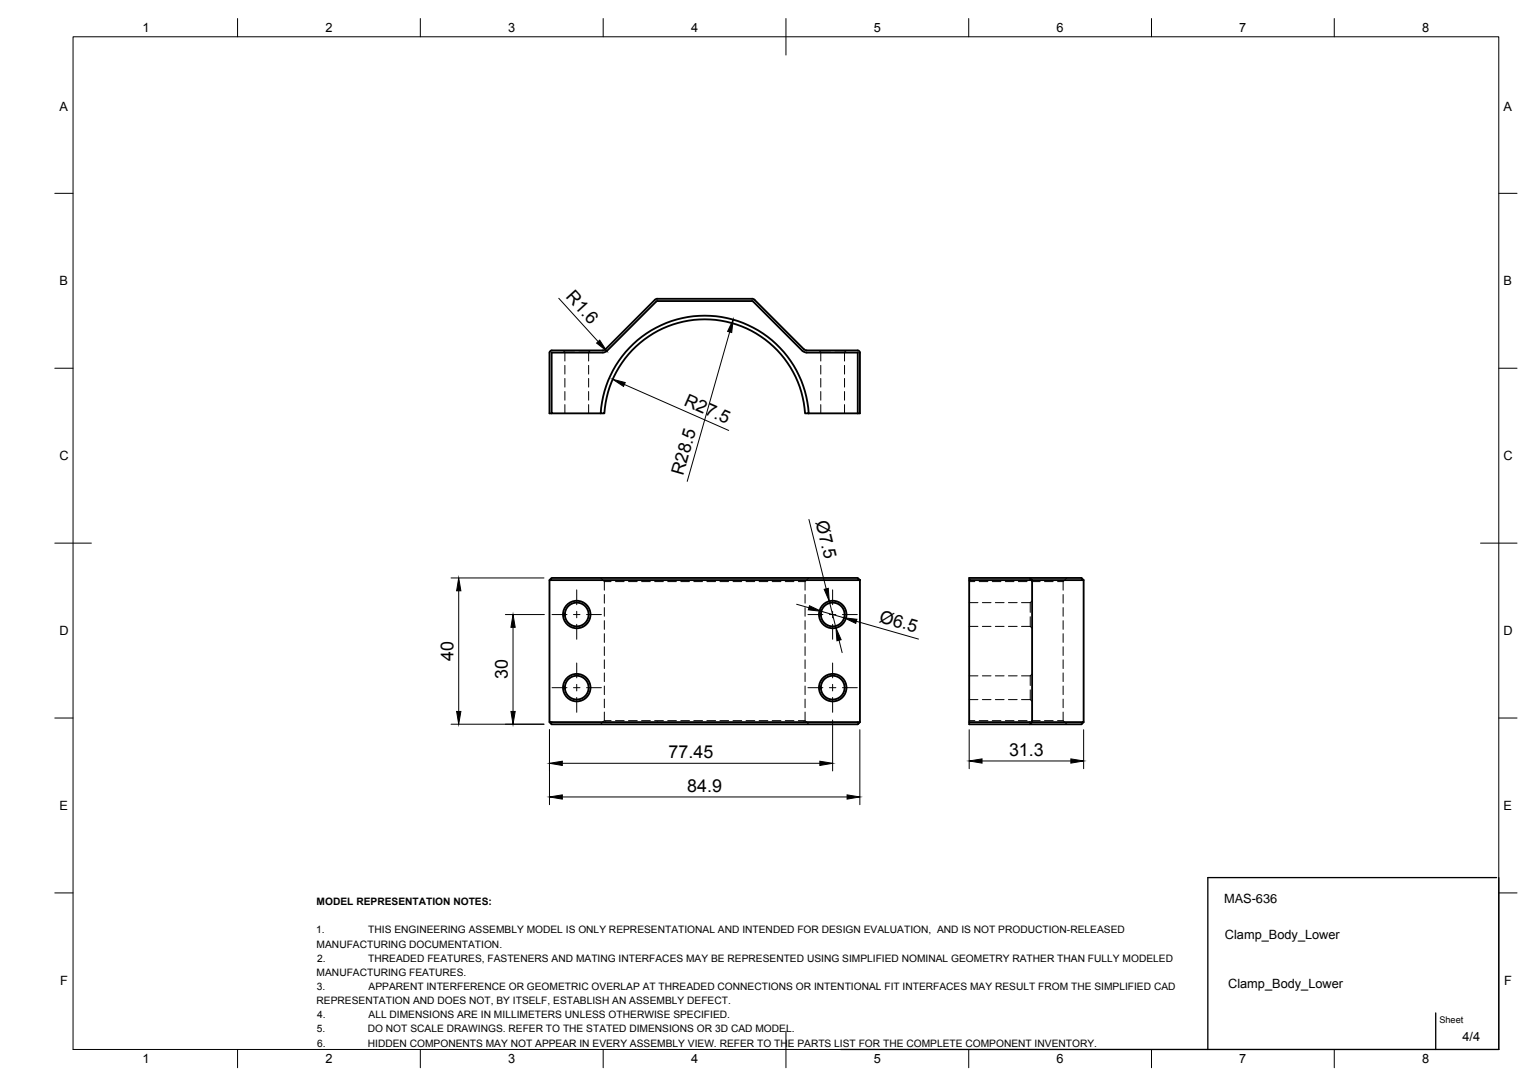
ISO-10303-21;
HEADER;
FILE_DESCRIPTION((''),'2;1');
FILE_NAME('Clamp_Body_Lower.step','2026-10-09T10:15:02-07:00',(''),(''),'','','');
FILE_SCHEMA (('AUTOMOTIVE_DESIGN { 1 0 10303 214 3 1 1 }'));
ENDSEC;
DATA;
#10=MECHANICAL_DESIGN_GEOMETRIC_PRESENTATION_REPRESENTATION('',(#84),#6779);
#59=B_SPLINE_CURVE_WITH_KNOTS('',3,(#6151,#6152,#6153,#6154),
 .UNSPECIFIED.,.F.,.F.,(4,4),(0.,2.0142284459),.UNSPECIFIED.) ;
#60=B_SPLINE_CURVE_WITH_KNOTS('',3,(#6158,#6159,#6160,#6161),
 .UNSPECIFIED.,.F.,.F.,(4,4),(0.,2.0142284459),.UNSPECIFIED.) ;
#61=B_SPLINE_CURVE_WITH_KNOTS('',3,(#6173,#6174,#6175,#6176),
 .UNSPECIFIED.,.F.,.F.,(4,4),(0.,2.0142284459),.UNSPECIFIED.) ;
#62=B_SPLINE_CURVE_WITH_KNOTS('',3,(#6177,#6178,#6179,#6180),
 .UNSPECIFIED.,.F.,.F.,(4,4),(0.,2.0142284459),.UNSPECIFIED.) ;
#64=SHAPE_REPRESENTATION_RELATIONSHIP('SRR','None',#6818,#74) ;
#74=ADVANCED_BREP_SHAPE_REPRESENTATION('',(#94),#6770) ;
#84=STYLED_ITEM('',(#6876),#94) ;
#94=MANIFOLD_SOLID_BREP('Body1',#3896) ;
#111=FACE_BOUND('',#719,.T.) ;
#112=FACE_BOUND('',#720,.T.) ;
#113=FACE_BOUND('',#722,.T.) ;
#114=FACE_BOUND('',#723,.T.) ;
#115=FACE_BOUND('',#745,.T.) ;
#116=FACE_BOUND('',#746,.T.) ;
#117=FACE_BOUND('',#752,.T.) ;
#118=FACE_BOUND('',#753,.T.) ;
#190=PLANE('',#4200) ;
#191=PLANE('',#4209) ;
#192=PLANE('',#4212) ;
#193=PLANE('',#4215) ;
#194=PLANE('',#4218) ;
#195=PLANE('',#4221) ;
#196=PLANE('',#4224) ;
#197=PLANE('',#4225) ;
#198=PLANE('',#4226) ;
#199=PLANE('',#4237) ;
#200=PLANE('',#4238) ;
#201=PLANE('',#4241) ;
#202=PLANE('',#4244) ;
#203=PLANE('',#4247) ;
#204=PLANE('',#4250) ;
#205=PLANE('',#4253) ;
#206=PLANE('',#4257) ;
#207=PLANE('',#4259) ;
#208=PLANE('',#4261) ;
#209=PLANE('',#4263) ;
#210=PLANE('',#4265) ;
#211=PLANE('',#4267) ;
#212=PLANE('',#4268) ;
#213=PLANE('',#4277) ;
#214=PLANE('',#4288) ;
#305=CONICAL_SURFACE('',#4193,1.,0.785398163397) ;
#306=CONICAL_SURFACE('',#4198,1.,0.785398163397) ;
#307=CONICAL_SURFACE('',#4207,1.,0.785398163397) ;
#308=CONICAL_SURFACE('',#4210,1.,0.785398163397) ;
#309=CONICAL_SURFACE('',#4213,1.,0.785398163397) ;
#310=CONICAL_SURFACE('',#4216,1.,0.785398163397) ;
#311=CONICAL_SURFACE('',#4219,1.,0.785398163397) ;
#312=CONICAL_SURFACE('',#4222,1.,0.785398163397) ;
#313=CONICAL_SURFACE('',#4256,1.,0.785398163397) ;
#314=CONICAL_SURFACE('',#4258,1.,0.785398163397) ;
#315=CONICAL_SURFACE('',#4260,1.,0.785398163397) ;
#316=CONICAL_SURFACE('',#4262,1.,0.785398163397) ;
#317=CONICAL_SURFACE('',#4264,1.,0.785398163397) ;
#318=CONICAL_SURFACE('',#4266,1.,0.785398163397) ;
#319=CONICAL_SURFACE('',#4272,1.,0.785398163398) ;
#320=CONICAL_SURFACE('',#4279,1.,0.785398163398) ;
#321=CONICAL_SURFACE('',#4283,1.,0.785398163398) ;
#322=CONICAL_SURFACE('',#4290,1.,0.785398163398) ;
#441=FACE_OUTER_BOUND('',#693,.T.) ;
#442=FACE_OUTER_BOUND('',#694,.T.) ;
#443=FACE_OUTER_BOUND('',#695,.T.) ;
#444=FACE_OUTER_BOUND('',#696,.T.) ;
#445=FACE_OUTER_BOUND('',#697,.T.) ;
#446=FACE_OUTER_BOUND('',#698,.T.) ;
#447=FACE_OUTER_BOUND('',#699,.T.) ;
#448=FACE_OUTER_BOUND('',#700,.T.) ;
#449=FACE_OUTER_BOUND('',#701,.T.) ;
#450=FACE_OUTER_BOUND('',#702,.T.) ;
#451=FACE_OUTER_BOUND('',#703,.T.) ;
#452=FACE_OUTER_BOUND('',#704,.T.) ;
#453=FACE_OUTER_BOUND('',#705,.T.) ;
#454=FACE_OUTER_BOUND('',#706,.T.) ;
#455=FACE_OUTER_BOUND('',#707,.T.) ;
#456=FACE_OUTER_BOUND('',#708,.T.) ;
#457=FACE_OUTER_BOUND('',#709,.T.) ;
#458=FACE_OUTER_BOUND('',#710,.T.) ;
#459=FACE_OUTER_BOUND('',#711,.T.) ;
#460=FACE_OUTER_BOUND('',#712,.T.) ;
#461=FACE_OUTER_BOUND('',#713,.T.) ;
#462=FACE_OUTER_BOUND('',#714,.T.) ;
#463=FACE_OUTER_BOUND('',#715,.T.) ;
#464=FACE_OUTER_BOUND('',#716,.T.) ;
#465=FACE_OUTER_BOUND('',#717,.T.) ;
#466=FACE_OUTER_BOUND('',#718,.T.) ;
#467=FACE_OUTER_BOUND('',#721,.T.) ;
#468=FACE_OUTER_BOUND('',#724,.T.) ;
#469=FACE_OUTER_BOUND('',#725,.T.) ;
#470=FACE_OUTER_BOUND('',#726,.T.) ;
#471=FACE_OUTER_BOUND('',#727,.T.) ;
#472=FACE_OUTER_BOUND('',#728,.T.) ;
#473=FACE_OUTER_BOUND('',#729,.T.) ;
#474=FACE_OUTER_BOUND('',#730,.T.) ;
#475=FACE_OUTER_BOUND('',#731,.T.) ;
#476=FACE_OUTER_BOUND('',#732,.T.) ;
#477=FACE_OUTER_BOUND('',#733,.T.) ;
#478=FACE_OUTER_BOUND('',#734,.T.) ;
#479=FACE_OUTER_BOUND('',#735,.T.) ;
#480=FACE_OUTER_BOUND('',#736,.T.) ;
#481=FACE_OUTER_BOUND('',#737,.T.) ;
#482=FACE_OUTER_BOUND('',#738,.T.) ;
#483=FACE_OUTER_BOUND('',#739,.T.) ;
#484=FACE_OUTER_BOUND('',#740,.T.) ;
#485=FACE_OUTER_BOUND('',#741,.T.) ;
#486=FACE_OUTER_BOUND('',#742,.T.) ;
#487=FACE_OUTER_BOUND('',#743,.T.) ;
#488=FACE_OUTER_BOUND('',#744,.T.) ;
#489=FACE_OUTER_BOUND('',#747,.T.) ;
#490=FACE_OUTER_BOUND('',#748,.T.) ;
#491=FACE_OUTER_BOUND('',#749,.T.) ;
#492=FACE_OUTER_BOUND('',#750,.T.) ;
#493=FACE_OUTER_BOUND('',#751,.T.) ;
#494=FACE_OUTER_BOUND('',#754,.T.) ;
#693=EDGE_LOOP('',(#3051,#3052,#3053,#3054)) ;
#694=EDGE_LOOP('',(#3055,#3056,#3057,#3058)) ;
#695=EDGE_LOOP('',(#3059,#3060,#3061,#3062)) ;
#696=EDGE_LOOP('',(#3063,#3064,#3065,#3066,#3067,#3068,#3069,#3070,#3071,
#3072,#3073,#3074,#3075,#3076,#3077,#3078)) ;
#697=EDGE_LOOP('',(#3079,#3080,#3081,#3082)) ;
#698=EDGE_LOOP('',(#3083,#3084,#3085,#3086)) ;
#699=EDGE_LOOP('',(#3087,#3088,#3089,#3090)) ;
#700=EDGE_LOOP('',(#3091,#3092,#3093,#3094)) ;
#701=EDGE_LOOP('',(#3095,#3096,#3097,#3098)) ;
#702=EDGE_LOOP('',(#3099,#3100,#3101,#3102)) ;
#703=EDGE_LOOP('',(#3103,#3104,#3105,#3106)) ;
#704=EDGE_LOOP('',(#3107,#3108,#3109,#3110)) ;
#705=EDGE_LOOP('',(#3111,#3112,#3113,#3114)) ;
#706=EDGE_LOOP('',(#3115,#3116,#3117,#3118)) ;
#707=EDGE_LOOP('',(#3119,#3120,#3121,#3122)) ;
#708=EDGE_LOOP('',(#3123,#3124,#3125,#3126)) ;
#709=EDGE_LOOP('',(#3127,#3128,#3129,#3130)) ;
#710=EDGE_LOOP('',(#3131,#3132,#3133,#3134,#3135,#3136,#3137,#3138,#3139,
#3140,#3141,#3142,#3143,#3144,#3145,#3146)) ;
#711=EDGE_LOOP('',(#3147,#3148,#3149,#3150)) ;
#712=EDGE_LOOP('',(#3151,#3152,#3153,#3154)) ;
#713=EDGE_LOOP('',(#3155,#3156,#3157,#3158)) ;
#714=EDGE_LOOP('',(#3159,#3160,#3161,#3162)) ;
#715=EDGE_LOOP('',(#3163,#3164,#3165,#3166)) ;
#716=EDGE_LOOP('',(#3167,#3168,#3169,#3170)) ;
#717=EDGE_LOOP('',(#3171,#3172,#3173,#3174)) ;
#718=EDGE_LOOP('',(#3175,#3176,#3177,#3178,#3179,#3180,#3181,#3182)) ;
#719=EDGE_LOOP('',(#3183)) ;
#720=EDGE_LOOP('',(#3184)) ;
#721=EDGE_LOOP('',(#3185,#3186,#3187,#3188,#3189,#3190,#3191,#3192)) ;
#722=EDGE_LOOP('',(#3193)) ;
#723=EDGE_LOOP('',(#3194)) ;
#724=EDGE_LOOP('',(#3195,#3196,#3197,#3198)) ;
#725=EDGE_LOOP('',(#3199,#3200,#3201,#3202)) ;
#726=EDGE_LOOP('',(#3203,#3204,#3205,#3206)) ;
#727=EDGE_LOOP('',(#3207,#3208,#3209,#3210)) ;
#728=EDGE_LOOP('',(#3211,#3212,#3213,#3214)) ;
#729=EDGE_LOOP('',(#3215,#3216,#3217,#3218)) ;
#730=EDGE_LOOP('',(#3219,#3220,#3221,#3222)) ;
#731=EDGE_LOOP('',(#3223,#3224,#3225,#3226)) ;
#732=EDGE_LOOP('',(#3227,#3228,#3229,#3230)) ;
#733=EDGE_LOOP('',(#3231,#3232,#3233,#3234)) ;
#734=EDGE_LOOP('',(#3235,#3236,#3237,#3238)) ;
#735=EDGE_LOOP('',(#3239,#3240,#3241,#3242)) ;
#736=EDGE_LOOP('',(#3243,#3244,#3245,#3246)) ;
#737=EDGE_LOOP('',(#3247,#3248,#3249,#3250)) ;
#738=EDGE_LOOP('',(#3251,#3252,#3253,#3254)) ;
#739=EDGE_LOOP('',(#3255,#3256,#3257,#3258)) ;
#740=EDGE_LOOP('',(#3259,#3260,#3261,#3262)) ;
#741=EDGE_LOOP('',(#3263,#3264,#3265,#3266,#3267)) ;
#742=EDGE_LOOP('',(#3268,#3269,#3270,#3271,#3272)) ;
#743=EDGE_LOOP('',(#3273,#3274,#3275,#3276,#3277)) ;
#744=EDGE_LOOP('',(#3278,#3279,#3280,#3281)) ;
#745=EDGE_LOOP('',(#3282)) ;
#746=EDGE_LOOP('',(#3283)) ;
#747=EDGE_LOOP('',(#3284,#3285,#3286,#3287,#3288)) ;
#748=EDGE_LOOP('',(#3289,#3290,#3291,#3292,#3293)) ;
#749=EDGE_LOOP('',(#3294,#3295,#3296,#3297,#3298)) ;
#750=EDGE_LOOP('',(#3299,#3300,#3301,#3302,#3303)) ;
#751=EDGE_LOOP('',(#3304,#3305,#3306,#3307)) ;
#752=EDGE_LOOP('',(#3308)) ;
#753=EDGE_LOOP('',(#3309)) ;
#754=EDGE_LOOP('',(#3310,#3311,#3312,#3313,#3314)) ;
#1031=LINE('',#6165,#1391) ;
#1032=LINE('',#6168,#1392) ;
#1033=LINE('',#6183,#1393) ;
#1034=LINE('',#6185,#1394) ;
#1035=LINE('',#6187,#1395) ;
#1036=LINE('',#6191,#1396) ;
#1037=LINE('',#6195,#1397) ;
#1038=LINE('',#6199,#1398) ;
#1039=LINE('',#6203,#1399) ;
#1040=LINE('',#6207,#1400) ;
#1041=LINE('',#6210,#1401) ;
#1042=LINE('',#6213,#1402) ;
#1043=LINE('',#6216,#1403) ;
#1044=LINE('',#6219,#1404) ;
#1045=LINE('',#6220,#1405) ;
#1046=LINE('',#6224,#1406) ;
#1047=LINE('',#6227,#1407) ;
#1048=LINE('',#6228,#1408) ;
#1049=LINE('',#6232,#1409) ;
#1050=LINE('',#6235,#1410) ;
#1051=LINE('',#6236,#1411) ;
#1052=LINE('',#6240,#1412) ;
#1053=LINE('',#6243,#1413) ;
#1054=LINE('',#6244,#1414) ;
#1055=LINE('',#6248,#1415) ;
#1056=LINE('',#6251,#1416) ;
#1057=LINE('',#6252,#1417) ;
#1058=LINE('',#6256,#1418) ;
#1059=LINE('',#6259,#1419) ;
#1060=LINE('',#6260,#1420) ;
#1061=LINE('',#6263,#1421) ;
#1062=LINE('',#6264,#1422) ;
#1063=LINE('',#6268,#1423) ;
#1064=LINE('',#6272,#1424) ;
#1065=LINE('',#6276,#1425) ;
#1066=LINE('',#6280,#1426) ;
#1067=LINE('',#6284,#1427) ;
#1068=LINE('',#6288,#1428) ;
#1069=LINE('',#6292,#1429) ;
#1070=LINE('',#6293,#1430) ;
#1071=LINE('',#6294,#1431) ;
#1072=LINE('',#6299,#1432) ;
#1073=LINE('',#6300,#1433) ;
#1074=LINE('',#6303,#1434) ;
#1075=LINE('',#6305,#1435) ;
#1076=LINE('',#6309,#1436) ;
#1077=LINE('',#6310,#1437) ;
#1078=LINE('',#6313,#1438) ;
#1079=LINE('',#6314,#1439) ;
#1080=LINE('',#6317,#1440) ;
#1081=LINE('',#6320,#1441) ;
#1082=LINE('',#6324,#1442) ;
#1083=LINE('',#6327,#1443) ;
#1084=LINE('',#6328,#1444) ;
#1085=LINE('',#6335,#1445) ;
#1086=LINE('',#6336,#1446) ;
#1087=LINE('',#6343,#1447) ;
#1088=LINE('',#6344,#1448) ;
#1089=LINE('',#6347,#1449) ;
#1090=LINE('',#6351,#1450) ;
#1091=LINE('',#6352,#1451) ;
#1092=LINE('',#6355,#1452) ;
#1093=LINE('',#6358,#1453) ;
#1094=LINE('',#6359,#1454) ;
#1095=LINE('',#6361,#1455) ;
#1096=LINE('',#6362,#1456) ;
#1097=LINE('',#6364,#1457) ;
#1098=LINE('',#6366,#1458) ;
#1099=LINE('',#6368,#1459) ;
#1100=LINE('',#6370,#1460) ;
#1101=LINE('',#6372,#1461) ;
#1102=LINE('',#6374,#1462) ;
#1103=LINE('',#6376,#1463) ;
#1104=LINE('',#6378,#1464) ;
#1105=LINE('',#6379,#1465) ;
#1106=LINE('',#6381,#1466) ;
#1107=LINE('',#6388,#1467) ;
#1108=LINE('',#6392,#1468) ;
#1109=LINE('',#6398,#1469) ;
#1110=LINE('',#6404,#1470) ;
#1111=LINE('',#6409,#1471) ;
#1112=LINE('',#6413,#1472) ;
#1113=LINE('',#6419,#1473) ;
#1114=LINE('',#6425,#1474) ;
#1391=VECTOR('',#4983,1.) ;
#1392=VECTOR('',#4986,1.) ;
#1393=VECTOR('',#4993,1.) ;
#1394=VECTOR('',#4994,1.) ;
#1395=VECTOR('',#4995,1.) ;
#1396=VECTOR('',#4998,1.) ;
#1397=VECTOR('',#5001,1.00000000000064) ;
#1398=VECTOR('',#5004,1.) ;
#1399=VECTOR('',#5007,1.00000000000064) ;
#1400=VECTOR('',#5010,1.) ;
#1401=VECTOR('',#5013,1.) ;
#1402=VECTOR('',#5016,1.00000000000064) ;
#1403=VECTOR('',#5019,1.00000000000064) ;
#1404=VECTOR('',#5022,1.) ;
#1405=VECTOR('',#5023,1.00000000000064) ;
#1406=VECTOR('',#5028,1.00000000000032) ;
#1407=VECTOR('',#5031,1.00000000000064) ;
#1408=VECTOR('',#5032,1.00000000000032) ;
#1409=VECTOR('',#5037,1.00000000000064) ;
#1410=VECTOR('',#5040,1.) ;
#1411=VECTOR('',#5041,1.00000000000064) ;
#1412=VECTOR('',#5046,1.00000000000032) ;
#1413=VECTOR('',#5049,1.00000000000064) ;
#1414=VECTOR('',#5050,1.00000000000032) ;
#1415=VECTOR('',#5055,1.00000000000064) ;
#1416=VECTOR('',#5058,1.) ;
#1417=VECTOR('',#5059,1.00000000000064) ;
#1418=VECTOR('',#5064,1.00000000000064) ;
#1419=VECTOR('',#5067,1.) ;
#1420=VECTOR('',#5068,1.00000000000064) ;
#1421=VECTOR('',#5071,1.00000000000064) ;
#1422=VECTOR('',#5072,1.) ;
#1423=VECTOR('',#5075,1.) ;
#1424=VECTOR('',#5078,1.) ;
#1425=VECTOR('',#5081,1.00000000000064) ;
#1426=VECTOR('',#5084,1.) ;
#1427=VECTOR('',#5087,1.00000000000064) ;
#1428=VECTOR('',#5090,1.) ;
#1429=VECTOR('',#5093,1.) ;
#1430=VECTOR('',#5094,1.) ;
#1431=VECTOR('',#5095,1.) ;
#1432=VECTOR('',#5100,1.) ;
#1433=VECTOR('',#5101,1.) ;
#1434=VECTOR('',#5104,1.) ;
#1435=VECTOR('',#5105,1.) ;
#1436=VECTOR('',#5110,1.) ;
#1437=VECTOR('',#5111,1.00000000000064) ;
#1438=VECTOR('',#5114,1.00000000000064) ;
#1439=VECTOR('',#5115,1.) ;
#1440=VECTOR('',#5118,1.) ;
#1441=VECTOR('',#5123,1.) ;
#1442=VECTOR('',#5128,1.) ;
#1443=VECTOR('',#5131,1.) ;
#1444=VECTOR('',#5132,1.00000000000064) ;
#1445=VECTOR('',#5139,1.) ;
#1446=VECTOR('',#5140,1.00000000000064) ;
#1447=VECTOR('',#5147,1.) ;
#1448=VECTOR('',#5148,1.) ;
#1449=VECTOR('',#5151,1.) ;
#1450=VECTOR('',#5156,1.) ;
#1451=VECTOR('',#5157,1.) ;
#1452=VECTOR('',#5160,1.) ;
#1453=VECTOR('',#5165,1.00000000000053) ;
#1454=VECTOR('',#5166,1.00000000000064) ;
#1455=VECTOR('',#5169,1.00000000000064) ;
#1456=VECTOR('',#5170,1.) ;
#1457=VECTOR('',#5173,1.00000000000032) ;
#1458=VECTOR('',#5176,1.00000000000032) ;
#1459=VECTOR('',#5179,1.00000000000064) ;
#1460=VECTOR('',#5182,1.00000000000064) ;
#1461=VECTOR('',#5185,1.00000000000032) ;
#1462=VECTOR('',#5188,1.00000000000032) ;
#1463=VECTOR('',#5191,1.00000000000064) ;
#1464=VECTOR('',#5194,1.00000000000064) ;
#1465=VECTOR('',#5195,1.) ;
#1466=VECTOR('',#5198,1.0000000000003) ;
#1467=VECTOR('',#5207,3.25) ;
#1468=VECTOR('',#5212,1.) ;
#1469=VECTOR('',#5219,3.25) ;
#1470=VECTOR('',#5228,1.) ;
#1471=VECTOR('',#5233,3.25) ;
#1472=VECTOR('',#5238,1.) ;
#1473=VECTOR('',#5245,3.25) ;
#1474=VECTOR('',#5254,1.) ;
#1627=CIRCLE('',#4194,27.5) ;
#1628=CIRCLE('',#4195,28.5) ;
#1629=CIRCLE('',#4197,27.5) ;
#1630=CIRCLE('',#4199,28.5) ;
#1631=CIRCLE('',#4201,0.03) ;
#1632=CIRCLE('',#4202,1.6) ;
#1633=CIRCLE('',#4203,0.4) ;
#1634=CIRCLE('',#4204,0.4) ;
#1635=CIRCLE('',#4205,1.6) ;
#1636=CIRCLE('',#4206,0.03) ;
#1637=CIRCLE('',#4208,0.63) ;
#1638=CIRCLE('',#4211,1.) ;
#1639=CIRCLE('',#4214,1.) ;
#1640=CIRCLE('',#4217,1.) ;
#1641=CIRCLE('',#4220,1.) ;
#1642=CIRCLE('',#4223,0.63) ;
#1643=CIRCLE('',#4227,0.03) ;
#1644=CIRCLE('',#4228,1.6) ;
#1645=CIRCLE('',#4229,0.4) ;
#1646=CIRCLE('',#4230,0.4) ;
#1647=CIRCLE('',#4231,1.6) ;
#1648=CIRCLE('',#4232,0.03) ;
#1649=CIRCLE('',#4234,1.) ;
#1650=CIRCLE('',#4236,1.) ;
#1651=CIRCLE('',#4240,1.) ;
#1652=CIRCLE('',#4243,1.) ;
#1653=CIRCLE('',#4245,3.25) ;
#1654=CIRCLE('',#4246,3.25) ;
#1655=CIRCLE('',#4248,3.25) ;
#1656=CIRCLE('',#4249,3.25) ;
#1657=CIRCLE('',#4252,0.63) ;
#1658=CIRCLE('',#4255,0.63) ;
#1659=CIRCLE('',#4270,3.25) ;
#1660=CIRCLE('',#4271,3.25) ;
#1661=CIRCLE('',#4273,3.75) ;
#1662=CIRCLE('',#4275,3.25) ;
#1663=CIRCLE('',#4276,3.25) ;
#1664=CIRCLE('',#4278,3.75) ;
#1665=CIRCLE('',#4281,3.25) ;
#1666=CIRCLE('',#4282,3.25) ;
#1667=CIRCLE('',#4284,3.75) ;
#1668=CIRCLE('',#4286,3.25) ;
#1669=CIRCLE('',#4287,3.25) ;
#1670=CIRCLE('',#4289,3.75) ;
#1859=VERTEX_POINT('',#6149) ;
#1860=VERTEX_POINT('',#6150) ;
#1861=VERTEX_POINT('',#6155) ;
#1862=VERTEX_POINT('',#6157) ;
#1863=VERTEX_POINT('',#6164) ;
#1864=VERTEX_POINT('',#6166) ;
#1865=VERTEX_POINT('',#6170) ;
#1866=VERTEX_POINT('',#6171) ;
#1867=VERTEX_POINT('',#6182) ;
#1868=VERTEX_POINT('',#6184) ;
#1869=VERTEX_POINT('',#6186) ;
#1870=VERTEX_POINT('',#6188) ;
#1871=VERTEX_POINT('',#6190) ;
#1872=VERTEX_POINT('',#6192) ;
#1873=VERTEX_POINT('',#6194) ;
#1874=VERTEX_POINT('',#6196) ;
#1875=VERTEX_POINT('',#6198) ;
#1876=VERTEX_POINT('',#6200) ;
#1877=VERTEX_POINT('',#6202) ;
#1878=VERTEX_POINT('',#6204) ;
#1879=VERTEX_POINT('',#6206) ;
#1880=VERTEX_POINT('',#6208) ;
#1881=VERTEX_POINT('',#6212) ;
#1882=VERTEX_POINT('',#6214) ;
#1883=VERTEX_POINT('',#6218) ;
#1884=VERTEX_POINT('',#6222) ;
#1885=VERTEX_POINT('',#6226) ;
#1886=VERTEX_POINT('',#6230) ;
#1887=VERTEX_POINT('',#6234) ;
#1888=VERTEX_POINT('',#6238) ;
#1889=VERTEX_POINT('',#6242) ;
#1890=VERTEX_POINT('',#6246) ;
#1891=VERTEX_POINT('',#6250) ;
#1892=VERTEX_POINT('',#6254) ;
#1893=VERTEX_POINT('',#6258) ;
#1894=VERTEX_POINT('',#6262) ;
#1895=VERTEX_POINT('',#6266) ;
#1896=VERTEX_POINT('',#6267) ;
#1897=VERTEX_POINT('',#6269) ;
#1898=VERTEX_POINT('',#6271) ;
#1899=VERTEX_POINT('',#6273) ;
#1900=VERTEX_POINT('',#6275) ;
#1901=VERTEX_POINT('',#6277) ;
#1902=VERTEX_POINT('',#6279) ;
#1903=VERTEX_POINT('',#6281) ;
#1904=VERTEX_POINT('',#6283) ;
#1905=VERTEX_POINT('',#6285) ;
#1906=VERTEX_POINT('',#6287) ;
#1907=VERTEX_POINT('',#6289) ;
#1908=VERTEX_POINT('',#6291) ;
#1909=VERTEX_POINT('',#6296) ;
#1910=VERTEX_POINT('',#6297) ;
#1911=VERTEX_POINT('',#6302) ;
#1912=VERTEX_POINT('',#6304) ;
#1913=VERTEX_POINT('',#6308) ;
#1914=VERTEX_POINT('',#6312) ;
#1915=VERTEX_POINT('',#6316) ;
#1916=VERTEX_POINT('',#6322) ;
#1917=VERTEX_POINT('',#6326) ;
#1918=VERTEX_POINT('',#6329) ;
#1919=VERTEX_POINT('',#6331) ;
#1920=VERTEX_POINT('',#6334) ;
#1921=VERTEX_POINT('',#6337) ;
#1922=VERTEX_POINT('',#6339) ;
#1923=VERTEX_POINT('',#6342) ;
#1924=VERTEX_POINT('',#6346) ;
#1925=VERTEX_POINT('',#6350) ;
#1926=VERTEX_POINT('',#6354) ;
#1927=VERTEX_POINT('',#6385) ;
#1928=VERTEX_POINT('',#6386) ;
#1929=VERTEX_POINT('',#6391) ;
#1930=VERTEX_POINT('',#6395) ;
#1931=VERTEX_POINT('',#6396) ;
#1932=VERTEX_POINT('',#6401) ;
#1933=VERTEX_POINT('',#6406) ;
#1934=VERTEX_POINT('',#6407) ;
#1935=VERTEX_POINT('',#6412) ;
#1936=VERTEX_POINT('',#6416) ;
#1937=VERTEX_POINT('',#6417) ;
#1938=VERTEX_POINT('',#6422) ;
#2279=EDGE_CURVE('',#1859,#1860,#59,.F.) ;
#2280=EDGE_CURVE('',#1861,#1860,#1627,.F.) ;
#2281=EDGE_CURVE('',#1861,#1862,#60,.T.) ;
#2282=EDGE_CURVE('',#1862,#1859,#1628,.F.) ;
#2283=EDGE_CURVE('',#1860,#1863,#1031,.T.) ;
#2284=EDGE_CURVE('',#1864,#1863,#1629,.F.) ;
#2285=EDGE_CURVE('',#1861,#1864,#1032,.T.) ;
#2286=EDGE_CURVE('',#1865,#1866,#1630,.F.) ;
#2287=EDGE_CURVE('',#1865,#1864,#61,.F.) ;
#2288=EDGE_CURVE('',#1863,#1866,#62,.T.) ;
#2289=EDGE_CURVE('',#1867,#1865,#1033,.F.) ;
#2290=EDGE_CURVE('',#1866,#1868,#1034,.T.) ;
#2291=EDGE_CURVE('',#1868,#1869,#1035,.F.) ;
#2292=EDGE_CURVE('',#1869,#1870,#1631,.T.) ;
#2293=EDGE_CURVE('',#1870,#1871,#1036,.F.) ;
#2294=EDGE_CURVE('',#1871,#1872,#1632,.F.) ;
#2295=EDGE_CURVE('',#1872,#1873,#1037,.F.) ;
#2296=EDGE_CURVE('',#1873,#1874,#1633,.T.) ;
#2297=EDGE_CURVE('',#1874,#1875,#1038,.F.) ;
#2298=EDGE_CURVE('',#1875,#1876,#1634,.T.) ;
#2299=EDGE_CURVE('',#1876,#1877,#1039,.T.) ;
#2300=EDGE_CURVE('',#1877,#1878,#1635,.F.) ;
#2301=EDGE_CURVE('',#1878,#1879,#1040,.F.) ;
#2302=EDGE_CURVE('',#1879,#1880,#1636,.T.) ;
#2303=EDGE_CURVE('',#1880,#1867,#1041,.T.) ;
#2304=EDGE_CURVE('',#1869,#1881,#1042,.T.) ;
#2305=EDGE_CURVE('',#1881,#1882,#1637,.T.) ;
#2306=EDGE_CURVE('',#1870,#1882,#1043,.T.) ;
#2307=EDGE_CURVE('',#1882,#1883,#1044,.F.) ;
#2308=EDGE_CURVE('',#1871,#1883,#1045,.F.) ;
#2309=EDGE_CURVE('',#1883,#1884,#1638,.F.) ;
#2310=EDGE_CURVE('',#1872,#1884,#1046,.F.) ;
#2311=EDGE_CURVE('',#1884,#1885,#1047,.F.) ;
#2312=EDGE_CURVE('',#1873,#1885,#1048,.F.) ;
#2313=EDGE_CURVE('',#1885,#1886,#1639,.T.) ;
#2314=EDGE_CURVE('',#1874,#1886,#1049,.T.) ;
#2315=EDGE_CURVE('',#1886,#1887,#1050,.F.) ;
#2316=EDGE_CURVE('',#1875,#1887,#1051,.F.) ;
#2317=EDGE_CURVE('',#1887,#1888,#1640,.T.) ;
#2318=EDGE_CURVE('',#1876,#1888,#1052,.T.) ;
#2319=EDGE_CURVE('',#1888,#1889,#1053,.T.) ;
#2320=EDGE_CURVE('',#1877,#1889,#1054,.F.) ;
#2321=EDGE_CURVE('',#1889,#1890,#1641,.F.) ;
#2322=EDGE_CURVE('',#1878,#1890,#1055,.F.) ;
#2323=EDGE_CURVE('',#1890,#1891,#1056,.F.) ;
#2324=EDGE_CURVE('',#1879,#1891,#1057,.F.) ;
#2325=EDGE_CURVE('',#1891,#1892,#1642,.T.) ;
#2326=EDGE_CURVE('',#1880,#1892,#1058,.T.) ;
#2327=EDGE_CURVE('',#1892,#1893,#1059,.T.) ;
#2328=EDGE_CURVE('',#1893,#1867,#1060,.T.) ;
#2329=EDGE_CURVE('',#1868,#1894,#1061,.F.) ;
#2330=EDGE_CURVE('',#1894,#1881,#1062,.F.) ;
#2331=EDGE_CURVE('',#1895,#1896,#1063,.T.) ;
#2332=EDGE_CURVE('',#1897,#1895,#1643,.T.) ;
#2333=EDGE_CURVE('',#1898,#1897,#1064,.F.) ;
#2334=EDGE_CURVE('',#1899,#1898,#1644,.F.) ;
#2335=EDGE_CURVE('',#1900,#1899,#1065,.T.) ;
#2336=EDGE_CURVE('',#1901,#1900,#1645,.T.) ;
#2337=EDGE_CURVE('',#1902,#1901,#1066,.F.) ;
#2338=EDGE_CURVE('',#1903,#1902,#1646,.T.) ;
#2339=EDGE_CURVE('',#1904,#1903,#1067,.F.) ;
#2340=EDGE_CURVE('',#1905,#1904,#1647,.F.) ;
#2341=EDGE_CURVE('',#1906,#1905,#1068,.F.) ;
#2342=EDGE_CURVE('',#1907,#1906,#1648,.T.) ;
#2343=EDGE_CURVE('',#1908,#1907,#1069,.F.) ;
#2344=EDGE_CURVE('',#1859,#1908,#1070,.T.) ;
#2345=EDGE_CURVE('',#1896,#1862,#1071,.F.) ;
#2346=EDGE_CURVE('',#1909,#1910,#1649,.F.) ;
#2347=EDGE_CURVE('',#1890,#1910,#1072,.F.) ;
#2348=EDGE_CURVE('',#1889,#1909,#1073,.F.) ;
#2349=EDGE_CURVE('',#1911,#1886,#1074,.T.) ;
#2350=EDGE_CURVE('',#1912,#1885,#1075,.T.) ;
#2351=EDGE_CURVE('',#1912,#1911,#1650,.T.) ;
#2352=EDGE_CURVE('',#1884,#1913,#1076,.F.) ;
#2353=EDGE_CURVE('',#1913,#1912,#1077,.F.) ;
#2354=EDGE_CURVE('',#1914,#1909,#1078,.T.) ;
#2355=EDGE_CURVE('',#1914,#1888,#1079,.T.) ;
#2356=EDGE_CURVE('',#1915,#1887,#1080,.T.) ;
#2357=EDGE_CURVE('',#1915,#1914,#1651,.T.) ;
#2358=EDGE_CURVE('',#1911,#1915,#1081,.F.) ;
#2359=EDGE_CURVE('',#1916,#1913,#1652,.F.) ;
#2360=EDGE_CURVE('',#1883,#1916,#1082,.F.) ;
#2361=EDGE_CURVE('',#1917,#1893,#1083,.T.) ;
#2362=EDGE_CURVE('',#1896,#1917,#1084,.F.) ;
#2363=EDGE_CURVE('',#1918,#1918,#1653,.T.) ;
#2364=EDGE_CURVE('',#1919,#1919,#1654,.T.) ;
#2365=EDGE_CURVE('',#1920,#1894,#1085,.T.) ;
#2366=EDGE_CURVE('',#1920,#1908,#1086,.T.) ;
#2367=EDGE_CURVE('',#1921,#1921,#1655,.T.) ;
#2368=EDGE_CURVE('',#1922,#1922,#1656,.T.) ;
#2369=EDGE_CURVE('',#1923,#1917,#1087,.T.) ;
#2370=EDGE_CURVE('',#1923,#1892,#1088,.T.) ;
#2371=EDGE_CURVE('',#1924,#1891,#1089,.T.) ;
#2372=EDGE_CURVE('',#1924,#1923,#1657,.T.) ;
#2373=EDGE_CURVE('',#1925,#1881,#1090,.T.) ;
#2374=EDGE_CURVE('',#1920,#1925,#1091,.F.) ;
#2375=EDGE_CURVE('',#1926,#1882,#1092,.T.) ;
#2376=EDGE_CURVE('',#1925,#1926,#1658,.T.) ;
#2377=EDGE_CURVE('',#1925,#1907,#1093,.F.) ;
#2378=EDGE_CURVE('',#1926,#1906,#1094,.F.) ;
#2379=EDGE_CURVE('',#1916,#1905,#1095,.T.) ;
#2380=EDGE_CURVE('',#1926,#1916,#1096,.F.) ;
#2381=EDGE_CURVE('',#1913,#1904,#1097,.T.) ;
#2382=EDGE_CURVE('',#1912,#1903,#1098,.T.) ;
#2383=EDGE_CURVE('',#1911,#1902,#1099,.F.) ;
#2384=EDGE_CURVE('',#1915,#1901,#1100,.T.) ;
#2385=EDGE_CURVE('',#1914,#1900,#1101,.F.) ;
#2386=EDGE_CURVE('',#1909,#1899,#1102,.T.) ;
#2387=EDGE_CURVE('',#1910,#1898,#1103,.T.) ;
#2388=EDGE_CURVE('',#1924,#1897,#1104,.T.) ;
#2389=EDGE_CURVE('',#1910,#1924,#1105,.F.) ;
#2390=EDGE_CURVE('',#1923,#1895,#1106,.F.) ;
#2391=EDGE_CURVE('',#1927,#1928,#1659,.F.) ;
#2392=EDGE_CURVE('',#1928,#1922,#1107,.T.) ;
#2393=EDGE_CURVE('',#1928,#1927,#1660,.F.) ;
#2394=EDGE_CURVE('',#1927,#1929,#1108,.T.) ;
#2395=EDGE_CURVE('',#1929,#1929,#1661,.T.) ;
#2396=EDGE_CURVE('',#1930,#1931,#1662,.F.) ;
#2397=EDGE_CURVE('',#1931,#1921,#1109,.T.) ;
#2398=EDGE_CURVE('',#1931,#1930,#1663,.F.) ;
#2399=EDGE_CURVE('',#1932,#1932,#1664,.T.) ;
#2400=EDGE_CURVE('',#1930,#1932,#1110,.T.) ;
#2401=EDGE_CURVE('',#1933,#1934,#1665,.F.) ;
#2402=EDGE_CURVE('',#1934,#1919,#1111,.T.) ;
#2403=EDGE_CURVE('',#1934,#1933,#1666,.F.) ;
#2404=EDGE_CURVE('',#1933,#1935,#1112,.T.) ;
#2405=EDGE_CURVE('',#1935,#1935,#1667,.T.) ;
#2406=EDGE_CURVE('',#1936,#1937,#1668,.F.) ;
#2407=EDGE_CURVE('',#1937,#1918,#1113,.T.) ;
#2408=EDGE_CURVE('',#1937,#1936,#1669,.F.) ;
#2409=EDGE_CURVE('',#1938,#1938,#1670,.T.) ;
#2410=EDGE_CURVE('',#1936,#1938,#1114,.T.) ;
#3051=ORIENTED_EDGE('',*,*,#2279,.T.) ;
#3052=ORIENTED_EDGE('',*,*,#2280,.F.) ;
#3053=ORIENTED_EDGE('',*,*,#2281,.T.) ;
#3054=ORIENTED_EDGE('',*,*,#2282,.T.) ;
#3055=ORIENTED_EDGE('',*,*,#2280,.T.) ;
#3056=ORIENTED_EDGE('',*,*,#2283,.T.) ;
#3057=ORIENTED_EDGE('',*,*,#2284,.F.) ;
#3058=ORIENTED_EDGE('',*,*,#2285,.F.) ;
#3059=ORIENTED_EDGE('',*,*,#2286,.F.) ;
#3060=ORIENTED_EDGE('',*,*,#2287,.T.) ;
#3061=ORIENTED_EDGE('',*,*,#2284,.T.) ;
#3062=ORIENTED_EDGE('',*,*,#2288,.T.) ;
#3063=ORIENTED_EDGE('',*,*,#2289,.T.) ;
#3064=ORIENTED_EDGE('',*,*,#2286,.T.) ;
#3065=ORIENTED_EDGE('',*,*,#2290,.T.) ;
#3066=ORIENTED_EDGE('',*,*,#2291,.T.) ;
#3067=ORIENTED_EDGE('',*,*,#2292,.T.) ;
#3068=ORIENTED_EDGE('',*,*,#2293,.T.) ;
#3069=ORIENTED_EDGE('',*,*,#2294,.T.) ;
#3070=ORIENTED_EDGE('',*,*,#2295,.T.) ;
#3071=ORIENTED_EDGE('',*,*,#2296,.T.) ;
#3072=ORIENTED_EDGE('',*,*,#2297,.T.) ;
#3073=ORIENTED_EDGE('',*,*,#2298,.T.) ;
#3074=ORIENTED_EDGE('',*,*,#2299,.T.) ;
#3075=ORIENTED_EDGE('',*,*,#2300,.T.) ;
#3076=ORIENTED_EDGE('',*,*,#2301,.T.) ;
#3077=ORIENTED_EDGE('',*,*,#2302,.T.) ;
#3078=ORIENTED_EDGE('',*,*,#2303,.T.) ;
#3079=ORIENTED_EDGE('',*,*,#2304,.T.) ;
#3080=ORIENTED_EDGE('',*,*,#2305,.T.) ;
#3081=ORIENTED_EDGE('',*,*,#2306,.F.) ;
#3082=ORIENTED_EDGE('',*,*,#2292,.F.) ;
#3083=ORIENTED_EDGE('',*,*,#2306,.T.) ;
#3084=ORIENTED_EDGE('',*,*,#2307,.T.) ;
#3085=ORIENTED_EDGE('',*,*,#2308,.F.) ;
#3086=ORIENTED_EDGE('',*,*,#2293,.F.) ;
#3087=ORIENTED_EDGE('',*,*,#2308,.T.) ;
#3088=ORIENTED_EDGE('',*,*,#2309,.T.) ;
#3089=ORIENTED_EDGE('',*,*,#2310,.F.) ;
#3090=ORIENTED_EDGE('',*,*,#2294,.F.) ;
#3091=ORIENTED_EDGE('',*,*,#2310,.T.) ;
#3092=ORIENTED_EDGE('',*,*,#2311,.T.) ;
#3093=ORIENTED_EDGE('',*,*,#2312,.F.) ;
#3094=ORIENTED_EDGE('',*,*,#2295,.F.) ;
#3095=ORIENTED_EDGE('',*,*,#2312,.T.) ;
#3096=ORIENTED_EDGE('',*,*,#2313,.T.) ;
#3097=ORIENTED_EDGE('',*,*,#2314,.F.) ;
#3098=ORIENTED_EDGE('',*,*,#2296,.F.) ;
#3099=ORIENTED_EDGE('',*,*,#2314,.T.) ;
#3100=ORIENTED_EDGE('',*,*,#2315,.T.) ;
#3101=ORIENTED_EDGE('',*,*,#2316,.F.) ;
#3102=ORIENTED_EDGE('',*,*,#2297,.F.) ;
#3103=ORIENTED_EDGE('',*,*,#2316,.T.) ;
#3104=ORIENTED_EDGE('',*,*,#2317,.T.) ;
#3105=ORIENTED_EDGE('',*,*,#2318,.F.) ;
#3106=ORIENTED_EDGE('',*,*,#2298,.F.) ;
#3107=ORIENTED_EDGE('',*,*,#2318,.T.) ;
#3108=ORIENTED_EDGE('',*,*,#2319,.T.) ;
#3109=ORIENTED_EDGE('',*,*,#2320,.F.) ;
#3110=ORIENTED_EDGE('',*,*,#2299,.F.) ;
#3111=ORIENTED_EDGE('',*,*,#2320,.T.) ;
#3112=ORIENTED_EDGE('',*,*,#2321,.T.) ;
#3113=ORIENTED_EDGE('',*,*,#2322,.F.) ;
#3114=ORIENTED_EDGE('',*,*,#2300,.F.) ;
#3115=ORIENTED_EDGE('',*,*,#2322,.T.) ;
#3116=ORIENTED_EDGE('',*,*,#2323,.T.) ;
#3117=ORIENTED_EDGE('',*,*,#2324,.F.) ;
#3118=ORIENTED_EDGE('',*,*,#2301,.F.) ;
#3119=ORIENTED_EDGE('',*,*,#2324,.T.) ;
#3120=ORIENTED_EDGE('',*,*,#2325,.T.) ;
#3121=ORIENTED_EDGE('',*,*,#2326,.F.) ;
#3122=ORIENTED_EDGE('',*,*,#2302,.F.) ;
#3123=ORIENTED_EDGE('',*,*,#2303,.F.) ;
#3124=ORIENTED_EDGE('',*,*,#2326,.T.) ;
#3125=ORIENTED_EDGE('',*,*,#2327,.T.) ;
#3126=ORIENTED_EDGE('',*,*,#2328,.T.) ;
#3127=ORIENTED_EDGE('',*,*,#2329,.T.) ;
#3128=ORIENTED_EDGE('',*,*,#2330,.T.) ;
#3129=ORIENTED_EDGE('',*,*,#2304,.F.) ;
#3130=ORIENTED_EDGE('',*,*,#2291,.F.) ;
#3131=ORIENTED_EDGE('',*,*,#2331,.F.) ;
#3132=ORIENTED_EDGE('',*,*,#2332,.F.) ;
#3133=ORIENTED_EDGE('',*,*,#2333,.F.) ;
#3134=ORIENTED_EDGE('',*,*,#2334,.F.) ;
#3135=ORIENTED_EDGE('',*,*,#2335,.F.) ;
#3136=ORIENTED_EDGE('',*,*,#2336,.F.) ;
#3137=ORIENTED_EDGE('',*,*,#2337,.F.) ;
#3138=ORIENTED_EDGE('',*,*,#2338,.F.) ;
#3139=ORIENTED_EDGE('',*,*,#2339,.F.) ;
#3140=ORIENTED_EDGE('',*,*,#2340,.F.) ;
#3141=ORIENTED_EDGE('',*,*,#2341,.F.) ;
#3142=ORIENTED_EDGE('',*,*,#2342,.F.) ;
#3143=ORIENTED_EDGE('',*,*,#2343,.F.) ;
#3144=ORIENTED_EDGE('',*,*,#2344,.F.) ;
#3145=ORIENTED_EDGE('',*,*,#2282,.F.) ;
#3146=ORIENTED_EDGE('',*,*,#2345,.F.) ;
#3147=ORIENTED_EDGE('',*,*,#2346,.T.) ;
#3148=ORIENTED_EDGE('',*,*,#2347,.F.) ;
#3149=ORIENTED_EDGE('',*,*,#2321,.F.) ;
#3150=ORIENTED_EDGE('',*,*,#2348,.T.) ;
#3151=ORIENTED_EDGE('',*,*,#2349,.T.) ;
#3152=ORIENTED_EDGE('',*,*,#2313,.F.) ;
#3153=ORIENTED_EDGE('',*,*,#2350,.F.) ;
#3154=ORIENTED_EDGE('',*,*,#2351,.T.) ;
#3155=ORIENTED_EDGE('',*,*,#2350,.T.) ;
#3156=ORIENTED_EDGE('',*,*,#2311,.F.) ;
#3157=ORIENTED_EDGE('',*,*,#2352,.T.) ;
#3158=ORIENTED_EDGE('',*,*,#2353,.T.) ;
#3159=ORIENTED_EDGE('',*,*,#2354,.T.) ;
#3160=ORIENTED_EDGE('',*,*,#2348,.F.) ;
#3161=ORIENTED_EDGE('',*,*,#2319,.F.) ;
#3162=ORIENTED_EDGE('',*,*,#2355,.F.) ;
#3163=ORIENTED_EDGE('',*,*,#2355,.T.) ;
#3164=ORIENTED_EDGE('',*,*,#2317,.F.) ;
#3165=ORIENTED_EDGE('',*,*,#2356,.F.) ;
#3166=ORIENTED_EDGE('',*,*,#2357,.T.) ;
#3167=ORIENTED_EDGE('',*,*,#2356,.T.) ;
#3168=ORIENTED_EDGE('',*,*,#2315,.F.) ;
#3169=ORIENTED_EDGE('',*,*,#2349,.F.) ;
#3170=ORIENTED_EDGE('',*,*,#2358,.T.) ;
#3171=ORIENTED_EDGE('',*,*,#2359,.T.) ;
#3172=ORIENTED_EDGE('',*,*,#2352,.F.) ;
#3173=ORIENTED_EDGE('',*,*,#2309,.F.) ;
#3174=ORIENTED_EDGE('',*,*,#2360,.T.) ;
#3175=ORIENTED_EDGE('',*,*,#2345,.T.) ;
#3176=ORIENTED_EDGE('',*,*,#2281,.F.) ;
#3177=ORIENTED_EDGE('',*,*,#2285,.T.) ;
#3178=ORIENTED_EDGE('',*,*,#2287,.F.) ;
#3179=ORIENTED_EDGE('',*,*,#2289,.F.) ;
#3180=ORIENTED_EDGE('',*,*,#2328,.F.) ;
#3181=ORIENTED_EDGE('',*,*,#2361,.F.) ;
#3182=ORIENTED_EDGE('',*,*,#2362,.F.) ;
#3183=ORIENTED_EDGE('',*,*,#2363,.F.) ;
#3184=ORIENTED_EDGE('',*,*,#2364,.F.) ;
#3185=ORIENTED_EDGE('',*,*,#2365,.T.) ;
#3186=ORIENTED_EDGE('',*,*,#2329,.F.) ;
#3187=ORIENTED_EDGE('',*,*,#2290,.F.) ;
#3188=ORIENTED_EDGE('',*,*,#2288,.F.) ;
#3189=ORIENTED_EDGE('',*,*,#2283,.F.) ;
#3190=ORIENTED_EDGE('',*,*,#2279,.F.) ;
#3191=ORIENTED_EDGE('',*,*,#2344,.T.) ;
#3192=ORIENTED_EDGE('',*,*,#2366,.F.) ;
#3193=ORIENTED_EDGE('',*,*,#2367,.F.) ;
#3194=ORIENTED_EDGE('',*,*,#2368,.F.) ;
#3195=ORIENTED_EDGE('',*,*,#2369,.T.) ;
#3196=ORIENTED_EDGE('',*,*,#2361,.T.) ;
#3197=ORIENTED_EDGE('',*,*,#2327,.F.) ;
#3198=ORIENTED_EDGE('',*,*,#2370,.F.) ;
#3199=ORIENTED_EDGE('',*,*,#2370,.T.) ;
#3200=ORIENTED_EDGE('',*,*,#2325,.F.) ;
#3201=ORIENTED_EDGE('',*,*,#2371,.F.) ;
#3202=ORIENTED_EDGE('',*,*,#2372,.T.) ;
#3203=ORIENTED_EDGE('',*,*,#2373,.T.) ;
#3204=ORIENTED_EDGE('',*,*,#2330,.F.) ;
#3205=ORIENTED_EDGE('',*,*,#2365,.F.) ;
#3206=ORIENTED_EDGE('',*,*,#2374,.T.) ;
#3207=ORIENTED_EDGE('',*,*,#2375,.T.) ;
#3208=ORIENTED_EDGE('',*,*,#2305,.F.) ;
#3209=ORIENTED_EDGE('',*,*,#2373,.F.) ;
#3210=ORIENTED_EDGE('',*,*,#2376,.T.) ;
#3211=ORIENTED_EDGE('',*,*,#2377,.T.) ;
#3212=ORIENTED_EDGE('',*,*,#2342,.T.) ;
#3213=ORIENTED_EDGE('',*,*,#2378,.F.) ;
#3214=ORIENTED_EDGE('',*,*,#2376,.F.) ;
#3215=ORIENTED_EDGE('',*,*,#2378,.T.) ;
#3216=ORIENTED_EDGE('',*,*,#2341,.T.) ;
#3217=ORIENTED_EDGE('',*,*,#2379,.F.) ;
#3218=ORIENTED_EDGE('',*,*,#2380,.F.) ;
#3219=ORIENTED_EDGE('',*,*,#2379,.T.) ;
#3220=ORIENTED_EDGE('',*,*,#2340,.T.) ;
#3221=ORIENTED_EDGE('',*,*,#2381,.F.) ;
#3222=ORIENTED_EDGE('',*,*,#2359,.F.) ;
#3223=ORIENTED_EDGE('',*,*,#2381,.T.) ;
#3224=ORIENTED_EDGE('',*,*,#2339,.T.) ;
#3225=ORIENTED_EDGE('',*,*,#2382,.F.) ;
#3226=ORIENTED_EDGE('',*,*,#2353,.F.) ;
#3227=ORIENTED_EDGE('',*,*,#2382,.T.) ;
#3228=ORIENTED_EDGE('',*,*,#2338,.T.) ;
#3229=ORIENTED_EDGE('',*,*,#2383,.F.) ;
#3230=ORIENTED_EDGE('',*,*,#2351,.F.) ;
#3231=ORIENTED_EDGE('',*,*,#2383,.T.) ;
#3232=ORIENTED_EDGE('',*,*,#2337,.T.) ;
#3233=ORIENTED_EDGE('',*,*,#2384,.F.) ;
#3234=ORIENTED_EDGE('',*,*,#2358,.F.) ;
#3235=ORIENTED_EDGE('',*,*,#2384,.T.) ;
#3236=ORIENTED_EDGE('',*,*,#2336,.T.) ;
#3237=ORIENTED_EDGE('',*,*,#2385,.F.) ;
#3238=ORIENTED_EDGE('',*,*,#2357,.F.) ;
#3239=ORIENTED_EDGE('',*,*,#2385,.T.) ;
#3240=ORIENTED_EDGE('',*,*,#2335,.T.) ;
#3241=ORIENTED_EDGE('',*,*,#2386,.F.) ;
#3242=ORIENTED_EDGE('',*,*,#2354,.F.) ;
#3243=ORIENTED_EDGE('',*,*,#2386,.T.) ;
#3244=ORIENTED_EDGE('',*,*,#2334,.T.) ;
#3245=ORIENTED_EDGE('',*,*,#2387,.F.) ;
#3246=ORIENTED_EDGE('',*,*,#2346,.F.) ;
#3247=ORIENTED_EDGE('',*,*,#2387,.T.) ;
#3248=ORIENTED_EDGE('',*,*,#2333,.T.) ;
#3249=ORIENTED_EDGE('',*,*,#2388,.F.) ;
#3250=ORIENTED_EDGE('',*,*,#2389,.F.) ;
#3251=ORIENTED_EDGE('',*,*,#2388,.T.) ;
#3252=ORIENTED_EDGE('',*,*,#2332,.T.) ;
#3253=ORIENTED_EDGE('',*,*,#2390,.F.) ;
#3254=ORIENTED_EDGE('',*,*,#2372,.F.) ;
#3255=ORIENTED_EDGE('',*,*,#2362,.T.) ;
#3256=ORIENTED_EDGE('',*,*,#2369,.F.) ;
#3257=ORIENTED_EDGE('',*,*,#2390,.T.) ;
#3258=ORIENTED_EDGE('',*,*,#2331,.T.) ;
#3259=ORIENTED_EDGE('',*,*,#2343,.T.) ;
#3260=ORIENTED_EDGE('',*,*,#2377,.F.) ;
#3261=ORIENTED_EDGE('',*,*,#2374,.F.) ;
#3262=ORIENTED_EDGE('',*,*,#2366,.T.) ;
#3263=ORIENTED_EDGE('',*,*,#2391,.T.) ;
#3264=ORIENTED_EDGE('',*,*,#2392,.T.) ;
#3265=ORIENTED_EDGE('',*,*,#2368,.T.) ;
#3266=ORIENTED_EDGE('',*,*,#2392,.F.) ;
#3267=ORIENTED_EDGE('',*,*,#2393,.T.) ;
#3268=ORIENTED_EDGE('',*,*,#2391,.F.) ;
#3269=ORIENTED_EDGE('',*,*,#2394,.T.) ;
#3270=ORIENTED_EDGE('',*,*,#2395,.T.) ;
#3271=ORIENTED_EDGE('',*,*,#2394,.F.) ;
#3272=ORIENTED_EDGE('',*,*,#2393,.F.) ;
#3273=ORIENTED_EDGE('',*,*,#2396,.T.) ;
#3274=ORIENTED_EDGE('',*,*,#2397,.T.) ;
#3275=ORIENTED_EDGE('',*,*,#2367,.T.) ;
#3276=ORIENTED_EDGE('',*,*,#2397,.F.) ;
#3277=ORIENTED_EDGE('',*,*,#2398,.T.) ;
#3278=ORIENTED_EDGE('',*,*,#2360,.F.) ;
#3279=ORIENTED_EDGE('',*,*,#2307,.F.) ;
#3280=ORIENTED_EDGE('',*,*,#2375,.F.) ;
#3281=ORIENTED_EDGE('',*,*,#2380,.T.) ;
#3282=ORIENTED_EDGE('',*,*,#2399,.F.) ;
#3283=ORIENTED_EDGE('',*,*,#2395,.F.) ;
#3284=ORIENTED_EDGE('',*,*,#2396,.F.) ;
#3285=ORIENTED_EDGE('',*,*,#2400,.T.) ;
#3286=ORIENTED_EDGE('',*,*,#2399,.T.) ;
#3287=ORIENTED_EDGE('',*,*,#2400,.F.) ;
#3288=ORIENTED_EDGE('',*,*,#2398,.F.) ;
#3289=ORIENTED_EDGE('',*,*,#2401,.T.) ;
#3290=ORIENTED_EDGE('',*,*,#2402,.T.) ;
#3291=ORIENTED_EDGE('',*,*,#2364,.T.) ;
#3292=ORIENTED_EDGE('',*,*,#2402,.F.) ;
#3293=ORIENTED_EDGE('',*,*,#2403,.T.) ;
#3294=ORIENTED_EDGE('',*,*,#2401,.F.) ;
#3295=ORIENTED_EDGE('',*,*,#2404,.T.) ;
#3296=ORIENTED_EDGE('',*,*,#2405,.T.) ;
#3297=ORIENTED_EDGE('',*,*,#2404,.F.) ;
#3298=ORIENTED_EDGE('',*,*,#2403,.F.) ;
#3299=ORIENTED_EDGE('',*,*,#2406,.T.) ;
#3300=ORIENTED_EDGE('',*,*,#2407,.T.) ;
#3301=ORIENTED_EDGE('',*,*,#2363,.T.) ;
#3302=ORIENTED_EDGE('',*,*,#2407,.F.) ;
#3303=ORIENTED_EDGE('',*,*,#2408,.T.) ;
#3304=ORIENTED_EDGE('',*,*,#2371,.T.) ;
#3305=ORIENTED_EDGE('',*,*,#2323,.F.) ;
#3306=ORIENTED_EDGE('',*,*,#2347,.T.) ;
#3307=ORIENTED_EDGE('',*,*,#2389,.T.) ;
#3308=ORIENTED_EDGE('',*,*,#2409,.F.) ;
#3309=ORIENTED_EDGE('',*,*,#2405,.F.) ;
#3310=ORIENTED_EDGE('',*,*,#2406,.F.) ;
#3311=ORIENTED_EDGE('',*,*,#2410,.T.) ;
#3312=ORIENTED_EDGE('',*,*,#2409,.T.) ;
#3313=ORIENTED_EDGE('',*,*,#2410,.F.) ;
#3314=ORIENTED_EDGE('',*,*,#2408,.F.) ;
#3624=CYLINDRICAL_SURFACE('',#4196,27.5) ;
#3625=CYLINDRICAL_SURFACE('',#4233,1.) ;
#3626=CYLINDRICAL_SURFACE('',#4235,1.) ;
#3627=CYLINDRICAL_SURFACE('',#4239,1.) ;
#3628=CYLINDRICAL_SURFACE('',#4242,1.) ;
#3629=CYLINDRICAL_SURFACE('',#4251,0.63) ;
#3630=CYLINDRICAL_SURFACE('',#4254,0.63) ;
#3631=CYLINDRICAL_SURFACE('',#4269,3.25) ;
#3632=CYLINDRICAL_SURFACE('',#4274,3.25) ;
#3633=CYLINDRICAL_SURFACE('',#4280,3.25) ;
#3634=CYLINDRICAL_SURFACE('',#4285,3.25) ;
#3765=ADVANCED_FACE('',(#441),#305,.F.) ;
#3766=ADVANCED_FACE('',(#442),#3624,.F.) ;
#3767=ADVANCED_FACE('',(#443),#306,.F.) ;
#3768=ADVANCED_FACE('',(#444),#190,.T.) ;
#3769=ADVANCED_FACE('',(#445),#307,.T.) ;
#3770=ADVANCED_FACE('',(#446),#191,.F.) ;
#3771=ADVANCED_FACE('',(#447),#308,.F.) ;
#3772=ADVANCED_FACE('',(#448),#192,.F.) ;
#3773=ADVANCED_FACE('',(#449),#309,.T.) ;
#3774=ADVANCED_FACE('',(#450),#193,.F.) ;
#3775=ADVANCED_FACE('',(#451),#310,.T.) ;
#3776=ADVANCED_FACE('',(#452),#194,.T.) ;
#3777=ADVANCED_FACE('',(#453),#311,.F.) ;
#3778=ADVANCED_FACE('',(#454),#195,.F.) ;
#3779=ADVANCED_FACE('',(#455),#312,.T.) ;
#3780=ADVANCED_FACE('',(#456),#196,.T.) ;
#3781=ADVANCED_FACE('',(#457),#197,.F.) ;
#3782=ADVANCED_FACE('',(#458),#198,.F.) ;
#3783=ADVANCED_FACE('',(#459),#3625,.F.) ;
#3784=ADVANCED_FACE('',(#460),#3626,.T.) ;
#3785=ADVANCED_FACE('',(#461),#199,.T.) ;
#3786=ADVANCED_FACE('',(#462),#200,.F.) ;
#3787=ADVANCED_FACE('',(#463),#3627,.T.) ;
#3788=ADVANCED_FACE('',(#464),#201,.T.) ;
#3789=ADVANCED_FACE('',(#465),#3628,.F.) ;
#3790=ADVANCED_FACE('',(#466,#111,#112),#202,.T.) ;
#3791=ADVANCED_FACE('',(#467,#113,#114),#203,.T.) ;
#3792=ADVANCED_FACE('',(#468),#204,.F.) ;
#3793=ADVANCED_FACE('',(#469),#3629,.T.) ;
#3794=ADVANCED_FACE('',(#470),#205,.T.) ;
#3795=ADVANCED_FACE('',(#471),#3630,.T.) ;
#3796=ADVANCED_FACE('',(#472),#313,.T.) ;
#3797=ADVANCED_FACE('',(#473),#206,.T.) ;
#3798=ADVANCED_FACE('',(#474),#314,.F.) ;
#3799=ADVANCED_FACE('',(#475),#207,.T.) ;
#3800=ADVANCED_FACE('',(#476),#315,.T.) ;
#3801=ADVANCED_FACE('',(#477),#208,.T.) ;
#3802=ADVANCED_FACE('',(#478),#316,.T.) ;
#3803=ADVANCED_FACE('',(#479),#209,.F.) ;
#3804=ADVANCED_FACE('',(#480),#317,.F.) ;
#3805=ADVANCED_FACE('',(#481),#210,.T.) ;
#3806=ADVANCED_FACE('',(#482),#318,.T.) ;
#3807=ADVANCED_FACE('',(#483),#211,.F.) ;
#3808=ADVANCED_FACE('',(#484),#212,.T.) ;
#3809=ADVANCED_FACE('',(#485),#3631,.F.) ;
#3810=ADVANCED_FACE('',(#486),#319,.F.) ;
#3811=ADVANCED_FACE('',(#487),#3632,.F.) ;
#3812=ADVANCED_FACE('',(#488,#115,#116),#213,.T.) ;
#3813=ADVANCED_FACE('',(#489),#320,.F.) ;
#3814=ADVANCED_FACE('',(#490),#3633,.F.) ;
#3815=ADVANCED_FACE('',(#491),#321,.F.) ;
#3816=ADVANCED_FACE('',(#492),#3634,.F.) ;
#3817=ADVANCED_FACE('',(#493,#117,#118),#214,.T.) ;
#3818=ADVANCED_FACE('',(#494),#322,.F.) ;
#3896=CLOSED_SHELL('',(#3765,#3766,#3767,#3768,#3769,#3770,#3771,#3772,
#3773,#3774,#3775,#3776,#3777,#3778,#3779,#3780,#3781,#3782,#3783,#3784,
#3785,#3786,#3787,#3788,#3789,#3790,#3791,#3792,#3793,#3794,#3795,#3796,
#3797,#3798,#3799,#3800,#3801,#3802,#3803,#3804,#3805,#3806,#3807,#3808,
#3809,#3810,#3811,#3812,#3813,#3814,#3815,#3816,#3817,#3818)) ;
#4192=AXIS2_PLACEMENT_3D('',#6147,#4973,#4974) ;
#4193=AXIS2_PLACEMENT_3D('',#6148,#4975,#4976) ;
#4194=AXIS2_PLACEMENT_3D('',#6156,#4977,#4978) ;
#4195=AXIS2_PLACEMENT_3D('',#6162,#4979,#4980) ;
#4196=AXIS2_PLACEMENT_3D('',#6163,#4981,#4982) ;
#4197=AXIS2_PLACEMENT_3D('',#6167,#4984,#4985) ;
#4198=AXIS2_PLACEMENT_3D('',#6169,#4987,#4988) ;
#4199=AXIS2_PLACEMENT_3D('',#6172,#4989,#4990) ;
#4200=AXIS2_PLACEMENT_3D('',#6181,#4991,#4992) ;
#4201=AXIS2_PLACEMENT_3D('',#6189,#4996,#4997) ;
#4202=AXIS2_PLACEMENT_3D('',#6193,#4999,#5000) ;
#4203=AXIS2_PLACEMENT_3D('',#6197,#5002,#5003) ;
#4204=AXIS2_PLACEMENT_3D('',#6201,#5005,#5006) ;
#4205=AXIS2_PLACEMENT_3D('',#6205,#5008,#5009) ;
#4206=AXIS2_PLACEMENT_3D('',#6209,#5011,#5012) ;
#4207=AXIS2_PLACEMENT_3D('',#6211,#5014,#5015) ;
#4208=AXIS2_PLACEMENT_3D('',#6215,#5017,#5018) ;
#4209=AXIS2_PLACEMENT_3D('',#6217,#5020,#5021) ;
#4210=AXIS2_PLACEMENT_3D('',#6221,#5024,#5025) ;
#4211=AXIS2_PLACEMENT_3D('',#6223,#5026,#5027) ;
#4212=AXIS2_PLACEMENT_3D('',#6225,#5029,#5030) ;
#4213=AXIS2_PLACEMENT_3D('',#6229,#5033,#5034) ;
#4214=AXIS2_PLACEMENT_3D('',#6231,#5035,#5036) ;
#4215=AXIS2_PLACEMENT_3D('',#6233,#5038,#5039) ;
#4216=AXIS2_PLACEMENT_3D('',#6237,#5042,#5043) ;
#4217=AXIS2_PLACEMENT_3D('',#6239,#5044,#5045) ;
#4218=AXIS2_PLACEMENT_3D('',#6241,#5047,#5048) ;
#4219=AXIS2_PLACEMENT_3D('',#6245,#5051,#5052) ;
#4220=AXIS2_PLACEMENT_3D('',#6247,#5053,#5054) ;
#4221=AXIS2_PLACEMENT_3D('',#6249,#5056,#5057) ;
#4222=AXIS2_PLACEMENT_3D('',#6253,#5060,#5061) ;
#4223=AXIS2_PLACEMENT_3D('',#6255,#5062,#5063) ;
#4224=AXIS2_PLACEMENT_3D('',#6257,#5065,#5066) ;
#4225=AXIS2_PLACEMENT_3D('',#6261,#5069,#5070) ;
#4226=AXIS2_PLACEMENT_3D('',#6265,#5073,#5074) ;
#4227=AXIS2_PLACEMENT_3D('',#6270,#5076,#5077) ;
#4228=AXIS2_PLACEMENT_3D('',#6274,#5079,#5080) ;
#4229=AXIS2_PLACEMENT_3D('',#6278,#5082,#5083) ;
#4230=AXIS2_PLACEMENT_3D('',#6282,#5085,#5086) ;
#4231=AXIS2_PLACEMENT_3D('',#6286,#5088,#5089) ;
#4232=AXIS2_PLACEMENT_3D('',#6290,#5091,#5092) ;
#4233=AXIS2_PLACEMENT_3D('',#6295,#5096,#5097) ;
#4234=AXIS2_PLACEMENT_3D('',#6298,#5098,#5099) ;
#4235=AXIS2_PLACEMENT_3D('',#6301,#5102,#5103) ;
#4236=AXIS2_PLACEMENT_3D('',#6306,#5106,#5107) ;
#4237=AXIS2_PLACEMENT_3D('',#6307,#5108,#5109) ;
#4238=AXIS2_PLACEMENT_3D('',#6311,#5112,#5113) ;
#4239=AXIS2_PLACEMENT_3D('',#6315,#5116,#5117) ;
#4240=AXIS2_PLACEMENT_3D('',#6318,#5119,#5120) ;
#4241=AXIS2_PLACEMENT_3D('',#6319,#5121,#5122) ;
#4242=AXIS2_PLACEMENT_3D('',#6321,#5124,#5125) ;
#4243=AXIS2_PLACEMENT_3D('',#6323,#5126,#5127) ;
#4244=AXIS2_PLACEMENT_3D('',#6325,#5129,#5130) ;
#4245=AXIS2_PLACEMENT_3D('',#6330,#5133,#5134) ;
#4246=AXIS2_PLACEMENT_3D('',#6332,#5135,#5136) ;
#4247=AXIS2_PLACEMENT_3D('',#6333,#5137,#5138) ;
#4248=AXIS2_PLACEMENT_3D('',#6338,#5141,#5142) ;
#4249=AXIS2_PLACEMENT_3D('',#6340,#5143,#5144) ;
#4250=AXIS2_PLACEMENT_3D('',#6341,#5145,#5146) ;
#4251=AXIS2_PLACEMENT_3D('',#6345,#5149,#5150) ;
#4252=AXIS2_PLACEMENT_3D('',#6348,#5152,#5153) ;
#4253=AXIS2_PLACEMENT_3D('',#6349,#5154,#5155) ;
#4254=AXIS2_PLACEMENT_3D('',#6353,#5158,#5159) ;
#4255=AXIS2_PLACEMENT_3D('',#6356,#5161,#5162) ;
#4256=AXIS2_PLACEMENT_3D('',#6357,#5163,#5164) ;
#4257=AXIS2_PLACEMENT_3D('',#6360,#5167,#5168) ;
#4258=AXIS2_PLACEMENT_3D('',#6363,#5171,#5172) ;
#4259=AXIS2_PLACEMENT_3D('',#6365,#5174,#5175) ;
#4260=AXIS2_PLACEMENT_3D('',#6367,#5177,#5178) ;
#4261=AXIS2_PLACEMENT_3D('',#6369,#5180,#5181) ;
#4262=AXIS2_PLACEMENT_3D('',#6371,#5183,#5184) ;
#4263=AXIS2_PLACEMENT_3D('',#6373,#5186,#5187) ;
#4264=AXIS2_PLACEMENT_3D('',#6375,#5189,#5190) ;
#4265=AXIS2_PLACEMENT_3D('',#6377,#5192,#5193) ;
#4266=AXIS2_PLACEMENT_3D('',#6380,#5196,#5197) ;
#4267=AXIS2_PLACEMENT_3D('',#6382,#5199,#5200) ;
#4268=AXIS2_PLACEMENT_3D('',#6383,#5201,#5202) ;
#4269=AXIS2_PLACEMENT_3D('',#6384,#5203,#5204) ;
#4270=AXIS2_PLACEMENT_3D('',#6387,#5205,#5206) ;
#4271=AXIS2_PLACEMENT_3D('',#6389,#5208,#5209) ;
#4272=AXIS2_PLACEMENT_3D('',#6390,#5210,#5211) ;
#4273=AXIS2_PLACEMENT_3D('',#6393,#5213,#5214) ;
#4274=AXIS2_PLACEMENT_3D('',#6394,#5215,#5216) ;
#4275=AXIS2_PLACEMENT_3D('',#6397,#5217,#5218) ;
#4276=AXIS2_PLACEMENT_3D('',#6399,#5220,#5221) ;
#4277=AXIS2_PLACEMENT_3D('',#6400,#5222,#5223) ;
#4278=AXIS2_PLACEMENT_3D('',#6402,#5224,#5225) ;
#4279=AXIS2_PLACEMENT_3D('',#6403,#5226,#5227) ;
#4280=AXIS2_PLACEMENT_3D('',#6405,#5229,#5230) ;
#4281=AXIS2_PLACEMENT_3D('',#6408,#5231,#5232) ;
#4282=AXIS2_PLACEMENT_3D('',#6410,#5234,#5235) ;
#4283=AXIS2_PLACEMENT_3D('',#6411,#5236,#5237) ;
#4284=AXIS2_PLACEMENT_3D('',#6414,#5239,#5240) ;
#4285=AXIS2_PLACEMENT_3D('',#6415,#5241,#5242) ;
#4286=AXIS2_PLACEMENT_3D('',#6418,#5243,#5244) ;
#4287=AXIS2_PLACEMENT_3D('',#6420,#5246,#5247) ;
#4288=AXIS2_PLACEMENT_3D('',#6421,#5248,#5249) ;
#4289=AXIS2_PLACEMENT_3D('',#6423,#5250,#5251) ;
#4290=AXIS2_PLACEMENT_3D('',#6424,#5252,#5253) ;
#4973=DIRECTION('axis',(0.,0.,1.)) ;
#4974=DIRECTION('refdir',(1.,0.,0.)) ;
#4975=DIRECTION('center_axis',(5.3290705182E-15,-7.9936057773E-15,-1.)) ;
#4976=DIRECTION('ref_axis',(1.38777878078155E-16,-1.,7.9936057773E-15)) ;
#4977=DIRECTION('center_axis',(2.11939249808E-15,3.56296341164E-15,1.)) ;
#4978=DIRECTION('ref_axis',(-1.,5.07218842173629E-46,2.11939249808E-15)) ;
#4979=DIRECTION('center_axis',(2.11939249808E-15,3.56296341164E-15,1.)) ;
#4980=DIRECTION('ref_axis',(-1.,5.07218842173629E-46,2.11939249808E-15)) ;
#4981=DIRECTION('center_axis',(0.,0.,1.)) ;
#4982=DIRECTION('ref_axis',(-0.997855551910869,-0.0654545454544914,0.)) ;
#4983=DIRECTION('',(0.,0.,1.)) ;
#4984=DIRECTION('center_axis',(0.,0.,1.)) ;
#4985=DIRECTION('ref_axis',(-1.,0.,0.)) ;
#4986=DIRECTION('',(0.,0.,1.)) ;
#4987=DIRECTION('center_axis',(5.3290705182E-15,-7.9936057773E-15,1.)) ;
#4988=DIRECTION('ref_axis',(-3.46944695195351E-16,-1.,-7.9936057773E-15)) ;
#4989=DIRECTION('center_axis',(-2.11939249808E-15,-3.56296341164E-15,1.)) ;
#4990=DIRECTION('ref_axis',(-1.,5.07218842173629E-46,-2.11939249808E-15)) ;
#4991=DIRECTION('center_axis',(0.,0.,1.)) ;
#4992=DIRECTION('ref_axis',(1.,0.,0.)) ;
#4993=DIRECTION('',(1.,0.,0.)) ;
#4994=DIRECTION('',(-1.,0.,0.)) ;
#4995=DIRECTION('',(0.,1.,0.)) ;
#4996=DIRECTION('center_axis',(0.,0.,1.)) ;
#4997=DIRECTION('ref_axis',(-1.,0.,0.)) ;
#4998=DIRECTION('',(-1.,0.,0.)) ;
#4999=DIRECTION('center_axis',(0.,0.,1.)) ;
#5000=DIRECTION('ref_axis',(-1.,0.,0.)) ;
#5001=DIRECTION('',(-0.707106781186548,0.707106781186548,0.)) ;
#5002=DIRECTION('center_axis',(0.,0.,1.)) ;
#5003=DIRECTION('ref_axis',(-1.,0.,0.)) ;
#5004=DIRECTION('',(-1.,0.,0.)) ;
#5005=DIRECTION('center_axis',(0.,0.,1.)) ;
#5006=DIRECTION('ref_axis',(-1.,0.,0.)) ;
#5007=DIRECTION('',(0.707106781186548,0.707106781186548,0.)) ;
#5008=DIRECTION('center_axis',(0.,0.,1.)) ;
#5009=DIRECTION('ref_axis',(-1.,0.,0.)) ;
#5010=DIRECTION('',(-1.,0.,0.)) ;
#5011=DIRECTION('center_axis',(0.,0.,1.)) ;
#5012=DIRECTION('ref_axis',(-1.,0.,0.)) ;
#5013=DIRECTION('',(0.,1.,0.)) ;
#5014=DIRECTION('center_axis',(0.,0.,-1.)) ;
#5015=DIRECTION('ref_axis',(-0.951056516295124,0.30901699437504,0.)) ;
#5016=DIRECTION('',(-0.707106781186548,4.18691322315732E-15,-0.707106781186548)) ;
#5017=DIRECTION('center_axis',(0.,0.,1.)) ;
#5018=DIRECTION('ref_axis',(-1.,0.,0.)) ;
#5019=DIRECTION('',(0.,-0.707106781186548,-0.707106781186548)) ;
#5020=DIRECTION('center_axis',(0.,0.707106781186548,-0.707106781186548)) ;
#5021=DIRECTION('ref_axis',(-1.,0.,0.)) ;
#5022=DIRECTION('',(-1.,0.,0.)) ;
#5023=DIRECTION('',(0.,0.707106781186548,0.707106781186548)) ;
#5024=DIRECTION('center_axis',(0.,-1.18423789293E-14,1.)) ;
#5025=DIRECTION('ref_axis',(0.968449269396153,0.249210779474039,2.95124848379779E-15)) ;
#5026=DIRECTION('center_axis',(2.85813443795E-15,-1.11068959943E-14,1.)) ;
#5027=DIRECTION('ref_axis',(-1.,1.53049221729886E-46,2.85813443795E-15)) ;
#5028=DIRECTION('',(0.49999999999984,0.49999999999984,0.707106781186774)) ;
#5029=DIRECTION('center_axis',(0.49999999999984,0.49999999999984,-0.707106781186774)) ;
#5030=DIRECTION('ref_axis',(-0.707106781186547,0.707106781186548,3.33066907361881E-16)) ;
#5031=DIRECTION('',(-0.707106781186548,0.707106781186548,0.)) ;
#5032=DIRECTION('',(0.49999999999984,0.49999999999984,0.707106781186774)) ;
#5033=DIRECTION('center_axis',(0.,0.,-1.)) ;
#5034=DIRECTION('ref_axis',(-0.770879376792195,-0.63698115077016,0.)) ;
#5035=DIRECTION('center_axis',(0.,0.,1.)) ;
#5036=DIRECTION('ref_axis',(-1.,0.,0.)) ;
#5037=DIRECTION('',(0.,-0.707106781186548,-0.707106781186548)) ;
#5038=DIRECTION('center_axis',(0.,0.707106781186548,-0.707106781186548)) ;
#5039=DIRECTION('ref_axis',(-1.,0.,0.)) ;
#5040=DIRECTION('',(-1.,0.,0.)) ;
#5041=DIRECTION('',(0.,0.707106781186548,0.707106781186548)) ;
#5042=DIRECTION('center_axis',(2.96059473233E-15,-1.18423789293E-14,-1.)) ;
#5043=DIRECTION('ref_axis',(-0.839857192231928,-0.542807421334954,3.94165438985342E-15)) ;
#5044=DIRECTION('center_axis',(-6.27102152096E-15,9.70281967417E-15,1.)) ;
#5045=DIRECTION('ref_axis',(-1.,-4.77240444652696E-45,-6.27102152096E-15)) ;
#5046=DIRECTION('',(0.49999999999984,-0.49999999999984,-0.707106781186774)) ;
#5047=DIRECTION('center_axis',(0.49999999999984,-0.49999999999984,0.707106781186774)) ;
#5048=DIRECTION('ref_axis',(0.707106781186547,0.707106781186548,3.33066907361881E-16)) ;
#5049=DIRECTION('',(0.707106781186548,0.707106781186548,0.)) ;
#5050=DIRECTION('',(-0.49999999999984,0.49999999999984,0.707106781186774)) ;
#5051=DIRECTION('center_axis',(-5.92118946467E-15,5.92118946467E-15,1.)) ;
#5052=DIRECTION('ref_axis',(0.097072775000982,0.995277286163815,-5.31843908861643E-15)) ;
#5053=DIRECTION('center_axis',(-6.43746510567E-15,6.27867841924E-16,1.)) ;
#5054=DIRECTION('ref_axis',(-1.,-2.64294780005913E-47,-6.43746510567E-15)) ;
#5055=DIRECTION('',(0.,0.707106781186548,0.707106781186548)) ;
#5056=DIRECTION('center_axis',(0.,0.707106781186548,-0.707106781186548)) ;
#5057=DIRECTION('ref_axis',(-1.,0.,0.)) ;
#5058=DIRECTION('',(-1.,0.,0.)) ;
#5059=DIRECTION('',(0.,0.707106781186548,0.707106781186548)) ;
#5060=DIRECTION('center_axis',(0.,0.,-1.)) ;
#5061=DIRECTION('ref_axis',(0.707106799571885,-0.70710676280121,0.)) ;
#5062=DIRECTION('center_axis',(0.,0.,1.)) ;
#5063=DIRECTION('ref_axis',(-1.,0.,0.)) ;
#5064=DIRECTION('',(0.707106781186548,-4.18691322315732E-15,-0.707106781186548)) ;
#5065=DIRECTION('center_axis',(0.707106781186548,0.,0.707106781186548)) ;
#5066=DIRECTION('ref_axis',(0.,1.,0.)) ;
#5067=DIRECTION('',(0.,1.,0.)) ;
#5068=DIRECTION('',(-0.707106781186548,0.,0.707106781186548)) ;
#5069=DIRECTION('center_axis',(0.707106781186548,0.,-0.707106781186548)) ;
#5070=DIRECTION('ref_axis',(0.,1.,0.)) ;
#5071=DIRECTION('',(0.707106781186548,0.,0.707106781186548)) ;
#5072=DIRECTION('',(0.,1.,0.)) ;
#5073=DIRECTION('center_axis',(0.,0.,1.)) ;
#5074=DIRECTION('ref_axis',(1.,0.,0.)) ;
#5075=DIRECTION('',(0.,1.,0.)) ;
#5076=DIRECTION('center_axis',(0.,0.,1.)) ;
#5077=DIRECTION('ref_axis',(-1.,0.,0.)) ;
#5078=DIRECTION('',(-1.,0.,0.)) ;
#5079=DIRECTION('center_axis',(0.,0.,1.)) ;
#5080=DIRECTION('ref_axis',(-1.,0.,0.)) ;
#5081=DIRECTION('',(0.707106781186548,0.707106781186548,0.)) ;
#5082=DIRECTION('center_axis',(0.,0.,1.)) ;
#5083=DIRECTION('ref_axis',(-1.,0.,0.)) ;
#5084=DIRECTION('',(-1.,0.,0.)) ;
#5085=DIRECTION('center_axis',(0.,0.,1.)) ;
#5086=DIRECTION('ref_axis',(-1.,0.,0.)) ;
#5087=DIRECTION('',(-0.707106781186548,0.707106781186548,0.)) ;
#5088=DIRECTION('center_axis',(0.,0.,1.)) ;
#5089=DIRECTION('ref_axis',(-1.,0.,0.)) ;
#5090=DIRECTION('',(-1.,0.,0.)) ;
#5091=DIRECTION('center_axis',(0.,0.,1.)) ;
#5092=DIRECTION('ref_axis',(-1.,0.,0.)) ;
#5093=DIRECTION('',(0.,1.,0.)) ;
#5094=DIRECTION('',(-1.,0.,0.)) ;
#5095=DIRECTION('',(1.,0.,0.)) ;
#5096=DIRECTION('center_axis',(0.,0.,1.)) ;
#5097=DIRECTION('ref_axis',(0.,1.,0.)) ;
#5098=DIRECTION('center_axis',(0.,0.,1.)) ;
#5099=DIRECTION('ref_axis',(-1.,0.,0.)) ;
#5100=DIRECTION('',(0.,0.,1.)) ;
#5101=DIRECTION('',(0.,0.,1.)) ;
#5102=DIRECTION('center_axis',(0.,0.,1.)) ;
#5103=DIRECTION('ref_axis',(-0.707106781186548,-0.707106781186548,0.)) ;
#5104=DIRECTION('',(0.,0.,1.)) ;
#5105=DIRECTION('',(0.,0.,1.)) ;
#5106=DIRECTION('center_axis',(0.,0.,1.)) ;
#5107=DIRECTION('ref_axis',(-1.,0.,0.)) ;
#5108=DIRECTION('center_axis',(-0.707106781186548,-0.707106781186548,0.)) ;
#5109=DIRECTION('ref_axis',(0.707106781186548,-0.707106781186548,0.)) ;
#5110=DIRECTION('',(0.,0.,1.)) ;
#5111=DIRECTION('',(-0.707106781186548,0.707106781186548,0.)) ;
#5112=DIRECTION('center_axis',(-0.707106781186548,0.707106781186548,0.)) ;
#5113=DIRECTION('ref_axis',(-0.707106781186548,-0.707106781186548,0.)) ;
#5114=DIRECTION('',(0.707106781186548,0.707106781186548,0.)) ;
#5115=DIRECTION('',(0.,0.,1.)) ;
#5116=DIRECTION('center_axis',(0.,0.,1.)) ;
#5117=DIRECTION('ref_axis',(1.11022302463E-16,-1.,0.)) ;
#5118=DIRECTION('',(0.,0.,1.)) ;
#5119=DIRECTION('center_axis',(0.,0.,1.)) ;
#5120=DIRECTION('ref_axis',(-1.,0.,0.)) ;
#5121=DIRECTION('center_axis',(0.,-1.,0.)) ;
#5122=DIRECTION('ref_axis',(1.,0.,0.)) ;
#5123=DIRECTION('',(-1.,0.,0.)) ;
#5124=DIRECTION('center_axis',(0.,0.,1.)) ;
#5125=DIRECTION('ref_axis',(0.707106781186548,0.707106781186548,0.)) ;
#5126=DIRECTION('center_axis',(0.,0.,1.)) ;
#5127=DIRECTION('ref_axis',(-1.,0.,0.)) ;
#5128=DIRECTION('',(0.,0.,1.)) ;
#5129=DIRECTION('center_axis',(0.,1.,0.)) ;
#5130=DIRECTION('ref_axis',(-1.,0.,0.)) ;
#5131=DIRECTION('',(0.,0.,1.)) ;
#5132=DIRECTION('',(-0.707106781186548,0.,-0.707106781186548)) ;
#5133=DIRECTION('center_axis',(0.,1.,0.)) ;
#5134=DIRECTION('ref_axis',(0.,0.,-1.)) ;
#5135=DIRECTION('center_axis',(0.,1.,0.)) ;
#5136=DIRECTION('ref_axis',(0.,0.,-1.)) ;
#5137=DIRECTION('center_axis',(0.,1.,0.)) ;
#5138=DIRECTION('ref_axis',(-1.,0.,0.)) ;
#5139=DIRECTION('',(0.,0.,1.)) ;
#5140=DIRECTION('',(0.707106781186548,0.,-0.707106781186548)) ;
#5141=DIRECTION('center_axis',(0.,1.,0.)) ;
#5142=DIRECTION('ref_axis',(0.,0.,-1.)) ;
#5143=DIRECTION('center_axis',(0.,1.,0.)) ;
#5144=DIRECTION('ref_axis',(0.,0.,-1.)) ;
#5145=DIRECTION('center_axis',(-1.,0.,0.)) ;
#5146=DIRECTION('ref_axis',(0.,-1.,0.)) ;
#5147=DIRECTION('',(0.,1.,0.)) ;
#5148=DIRECTION('',(0.,0.,1.)) ;
#5149=DIRECTION('center_axis',(0.,0.,1.)) ;
#5150=DIRECTION('ref_axis',(1.13626224362E-14,-1.,0.)) ;
#5151=DIRECTION('',(0.,0.,1.)) ;
#5152=DIRECTION('center_axis',(0.,0.,1.)) ;
#5153=DIRECTION('ref_axis',(-1.,0.,0.)) ;
#5154=DIRECTION('center_axis',(-1.,0.,0.)) ;
#5155=DIRECTION('ref_axis',(0.,-1.,0.)) ;
#5156=DIRECTION('',(0.,0.,1.)) ;
#5157=DIRECTION('',(0.,1.,0.)) ;
#5158=DIRECTION('center_axis',(0.,0.,1.)) ;
#5159=DIRECTION('ref_axis',(-1.,1.83697019872E-16,0.)) ;
#5160=DIRECTION('',(0.,0.,1.)) ;
#5161=DIRECTION('center_axis',(0.,0.,1.)) ;
#5162=DIRECTION('ref_axis',(-1.,0.,0.)) ;
#5163=DIRECTION('center_axis',(0.,0.,1.)) ;
#5164=DIRECTION('ref_axis',(-0.951056516295124,0.30901699437504,0.)) ;
#5165=DIRECTION('',(-0.707106780871626,2.11010493413889E-5,0.707106781186626)) ;
#5166=DIRECTION('',(0.,-0.707106781186548,0.707106781186548)) ;
#5167=DIRECTION('center_axis',(0.,-0.707106781186548,-0.707106781186548)) ;
#5168=DIRECTION('ref_axis',(-1.,0.,0.)) ;
#5169=DIRECTION('',(0.,0.707106781186548,-0.707106781186548)) ;
#5170=DIRECTION('',(-1.,0.,0.)) ;
#5171=DIRECTION('center_axis',(0.,-1.18423789293E-14,-1.)) ;
#5172=DIRECTION('ref_axis',(0.968449269396153,0.249210779474039,-2.95124848379779E-15)) ;
#5173=DIRECTION('',(0.49999999999984,0.49999999999984,-0.707106781186774)) ;
#5174=DIRECTION('center_axis',(-0.49999999999984,-0.49999999999984,-0.707106781186774)) ;
#5175=DIRECTION('ref_axis',(-0.707106781186547,0.707106781186548,-3.33066907361881E-16)) ;
#5176=DIRECTION('',(0.49999999999984,0.49999999999984,-0.707106781186774)) ;
#5177=DIRECTION('center_axis',(0.,0.,1.)) ;
#5178=DIRECTION('ref_axis',(-0.770879376792195,-0.63698115077016,0.)) ;
#5179=DIRECTION('',(0.,-0.707106781186548,0.707106781186548)) ;
#5180=DIRECTION('center_axis',(0.,-0.707106781186548,-0.707106781186548)) ;
#5181=DIRECTION('ref_axis',(-1.,0.,0.)) ;
#5182=DIRECTION('',(0.,0.707106781186548,-0.707106781186548)) ;
#5183=DIRECTION('center_axis',(2.96059473233E-15,-1.18423789293E-14,1.)) ;
#5184=DIRECTION('ref_axis',(-0.839857192231928,-0.542807421334954,-3.94165438985342E-15)) ;
#5185=DIRECTION('',(0.50000001947084,-0.49999998052884,0.707106781186774)) ;
#5186=DIRECTION('center_axis',(-0.49999999999984,0.49999999999984,0.707106781186774)) ;
#5187=DIRECTION('ref_axis',(0.707106781186547,0.707106781186548,-3.33066907361881E-16)) ;
#5188=DIRECTION('',(-0.49999999999984,0.49999999999984,-0.707106781186774)) ;
#5189=DIRECTION('center_axis',(-5.92118946467E-15,5.92118946467E-15,-1.)) ;
#5190=DIRECTION('ref_axis',(0.097072775000982,0.995277286163815,5.31843908861643E-15)) ;
#5191=DIRECTION('',(-4.28670243814725E-8,0.707106781186547,-0.707106781186547)) ;
#5192=DIRECTION('center_axis',(0.,-0.707106781186548,-0.707106781186548)) ;
#5193=DIRECTION('ref_axis',(-1.,0.,0.)) ;
#5194=DIRECTION('',(0.,0.707106781186548,-0.707106781186548)) ;
#5195=DIRECTION('',(-1.,0.,0.)) ;
#5196=DIRECTION('center_axis',(0.,0.,1.)) ;
#5197=DIRECTION('ref_axis',(0.707118857908102,-0.70709470425873,0.)) ;
#5198=DIRECTION('',(0.707106780773791,2.41533135191928E-5,0.707106781186791)) ;
#5199=DIRECTION('center_axis',(-0.707106781186548,0.,0.707106781186548)) ;
#5200=DIRECTION('ref_axis',(0.,1.,0.)) ;
#5201=DIRECTION('center_axis',(-0.707106781186548,0.,-0.707106781186548)) ;
#5202=DIRECTION('ref_axis',(0.,1.,0.)) ;
#5203=DIRECTION('center_axis',(0.,1.,0.)) ;
#5204=DIRECTION('ref_axis',(0.877582561890372,0.,-0.479425538604204)) ;
#5205=DIRECTION('center_axis',(0.,1.,0.)) ;
#5206=DIRECTION('ref_axis',(0.,0.,-1.)) ;
#5207=DIRECTION('',(0.,1.,0.)) ;
#5208=DIRECTION('center_axis',(0.,1.,0.)) ;
#5209=DIRECTION('ref_axis',(0.,0.,-1.)) ;
#5210=DIRECTION('center_axis',(1.42108547152E-14,-1.,3.16191517413E-13)) ;
#5211=DIRECTION('ref_axis',(-0.811184158891276,1.73378264946965E-13,0.584790783412199)) ;
#5212=DIRECTION('',(0.573593819543454,-0.70710678118628,-0.413509528526164)) ;
#5213=DIRECTION('center_axis',(1.54852556736E-13,-1.,2.14801506028E-13)) ;
#5214=DIRECTION('ref_axis',(4.47622740477785E-43,2.14801506028E-13,1.)) ;
#5215=DIRECTION('center_axis',(0.,1.,0.)) ;
#5216=DIRECTION('ref_axis',(0.877582561890372,0.,-0.479425538604204)) ;
#5217=DIRECTION('center_axis',(0.,1.,0.)) ;
#5218=DIRECTION('ref_axis',(0.,0.,-1.)) ;
#5219=DIRECTION('',(0.,1.,0.)) ;
#5220=DIRECTION('center_axis',(0.,1.,0.)) ;
#5221=DIRECTION('ref_axis',(0.,0.,-1.)) ;
#5222=DIRECTION('center_axis',(0.,-1.,0.)) ;
#5223=DIRECTION('ref_axis',(1.,0.,0.)) ;
#5224=DIRECTION('center_axis',(0.,-1.,0.)) ;
#5225=DIRECTION('ref_axis',(0.,0.,1.)) ;
#5226=DIRECTION('center_axis',(2.84217094304E-14,-1.,3.19744231092E-13)) ;
#5227=DIRECTION('ref_axis',(-0.811184158893383,1.63928238932276E-13,0.584790783409276)) ;
#5228=DIRECTION('',(0.573593819544954,-0.707106781186273,-0.413509528524095)) ;
#5229=DIRECTION('center_axis',(0.,1.,0.)) ;
#5230=DIRECTION('ref_axis',(0.877582561890372,0.,-0.479425538604204)) ;
#5231=DIRECTION('center_axis',(0.,1.,0.)) ;
#5232=DIRECTION('ref_axis',(0.,0.,-1.)) ;
#5233=DIRECTION('',(0.,1.,0.)) ;
#5234=DIRECTION('center_axis',(0.,1.,0.)) ;
#5235=DIRECTION('ref_axis',(0.,0.,-1.)) ;
#5236=DIRECTION('center_axis',(2.84217094304E-14,-1.,3.23296944771E-13)) ;
#5237=DIRECTION('ref_axis',(-0.811184158891618,1.66005833148689E-13,0.584790783411725)) ;
#5238=DIRECTION('',(0.573593819543705,-0.707106781186275,-0.413509528525824)) ;
#5239=DIRECTION('center_axis',(1.63083011564E-13,-1.,2.26218263553E-13)) ;
#5240=DIRECTION('ref_axis',(1.41626863241979E-42,2.26218263553E-13,1.)) ;
#5241=DIRECTION('center_axis',(0.,1.,0.)) ;
#5242=DIRECTION('ref_axis',(0.877582561890372,0.,-0.479425538604204)) ;
#5243=DIRECTION('center_axis',(0.,1.,0.)) ;
#5244=DIRECTION('ref_axis',(0.,0.,-1.)) ;
#5245=DIRECTION('',(0.,1.,0.)) ;
#5246=DIRECTION('center_axis',(0.,1.,0.)) ;
#5247=DIRECTION('ref_axis',(0.,0.,-1.)) ;
#5248=DIRECTION('center_axis',(0.,-1.,0.)) ;
#5249=DIRECTION('ref_axis',(1.,0.,0.)) ;
#5250=DIRECTION('center_axis',(0.,-1.,0.)) ;
#5251=DIRECTION('ref_axis',(0.,0.,1.)) ;
#5252=DIRECTION('center_axis',(4.26325641456E-14,-1.,3.23296944771E-13)) ;
#5253=DIRECTION('ref_axis',(-0.811184158884955,1.54478212922681E-13,0.584790783420967)) ;
#5254=DIRECTION('',(0.573593819539004,-0.707106781186267,-0.413509528532359)) ;
#6147=CARTESIAN_POINT('',(0.,0.,0.)) ;
#6148=CARTESIAN_POINT('Origin',(-1.46549439250795E-13,2.15383266777693E-13,
7.4999999999991)) ;
#6149=CARTESIAN_POINT('',(-28.4431010968,-1.8,-20.)) ;
#6150=CARTESIAN_POINT('',(-27.4410276775,-1.8,-19.)) ;
#6151=CARTESIAN_POINT('Ctrl Pts',(-27.4410276775,-1.8,-19.)) ;
#6152=CARTESIAN_POINT('Ctrl Pts',(-27.7749094354,-1.8,-19.3331657657)) ;
#6153=CARTESIAN_POINT('Ctrl Pts',(-28.108944209,-1.8,-19.6665102407)) ;
#6154=CARTESIAN_POINT('Ctrl Pts',(-28.4431010968,-1.8,-20.)) ;
#6155=CARTESIAN_POINT('',(27.4410276775,-1.8,-19.)) ;
#6156=CARTESIAN_POINT('Origin',(-5.3290705182E-15,3.5527136788E-15,-19.)) ;
#6157=CARTESIAN_POINT('',(28.4431010968,-1.8,-20.)) ;
#6158=CARTESIAN_POINT('Ctrl Pts',(27.4410276775,-1.8,-19.)) ;
#6159=CARTESIAN_POINT('Ctrl Pts',(27.7749094354,-1.8,-19.3331657657)) ;
#6160=CARTESIAN_POINT('Ctrl Pts',(28.108944209,-1.8,-19.6665102407)) ;
#6161=CARTESIAN_POINT('Ctrl Pts',(28.4431010968,-1.8,-20.)) ;
#6162=CARTESIAN_POINT('Origin',(-1.28742099732E-27,-4.4408920985E-15,-20.)) ;
#6163=CARTESIAN_POINT('Origin',(0.,0.,0.)) ;
#6164=CARTESIAN_POINT('',(-27.4410276775,-1.8,19.)) ;
#6165=CARTESIAN_POINT('',(-27.4410276775,-1.8,0.)) ;
#6166=CARTESIAN_POINT('',(27.4410276775,-1.8,19.)) ;
#6167=CARTESIAN_POINT('Origin',(0.,0.,19.)) ;
#6168=CARTESIAN_POINT('',(27.4410276775,-1.8,0.)) ;
#6169=CARTESIAN_POINT('Origin',(-1.46549439250795E-13,2.15383266777693E-13,
-7.4999999999991)) ;
#6170=CARTESIAN_POINT('',(28.4431010968,-1.8,20.)) ;
#6171=CARTESIAN_POINT('',(-28.4431010968,-1.8,20.)) ;
#6172=CARTESIAN_POINT('Origin',(-1.28742099732E-27,-4.4408920985E-15,20.)) ;
#6173=CARTESIAN_POINT('Ctrl Pts',(27.4410276775,-1.8,19.)) ;
#6174=CARTESIAN_POINT('Ctrl Pts',(27.7749094354,-1.8,19.3331657657)) ;
#6175=CARTESIAN_POINT('Ctrl Pts',(28.108944209,-1.8,19.6665102407)) ;
#6176=CARTESIAN_POINT('Ctrl Pts',(28.4431010968,-1.8,20.)) ;
#6177=CARTESIAN_POINT('Ctrl Pts',(-27.4410276775,-1.8,19.)) ;
#6178=CARTESIAN_POINT('Ctrl Pts',(-27.7749094354,-1.8,19.3331657657)) ;
#6179=CARTESIAN_POINT('Ctrl Pts',(-28.108944209,-1.8,19.6665102407)) ;
#6180=CARTESIAN_POINT('Ctrl Pts',(-28.4431010968,-1.8,20.)) ;
#6181=CARTESIAN_POINT('Origin',(0.,0.,20.)) ;
#6182=CARTESIAN_POINT('',(41.85,-1.8,20.)) ;
#6183=CARTESIAN_POINT('',(35.1465505484,-1.8,20.)) ;
#6184=CARTESIAN_POINT('',(-41.85,-1.8,20.)) ;
#6185=CARTESIAN_POINT('',(-35.1465505484,-1.8,20.)) ;
#6186=CARTESIAN_POINT('',(-41.85,-18.3699999990914,20.)) ;
#6187=CARTESIAN_POINT('',(-41.85,-10.085,20.)) ;
#6188=CARTESIAN_POINT('',(-41.82,-18.4,20.)) ;
#6189=CARTESIAN_POINT('Origin',(-41.82,-18.37,20.)) ;
#6190=CARTESIAN_POINT('',(-27.8642135633724,-18.4,20.)) ;
#6191=CARTESIAN_POINT('',(-34.8421067812,-18.4,20.)) ;
#6192=CARTESIAN_POINT('',(-26.7328427125,-18.8686291501,20.)) ;
#6193=CARTESIAN_POINT('Origin',(-27.8642135624,-20.,20.)) ;
#6194=CARTESIAN_POINT('',(-13.2186291495519,-32.382842713025,20.0000000000016)) ;
#6195=CARTESIAN_POINT('',(-19.9757359313,-25.6257359313,20.)) ;
#6196=CARTESIAN_POINT('',(-12.9357864376,-32.5,20.)) ;
#6197=CARTESIAN_POINT('Origin',(-12.9357864376,-32.1,20.)) ;
#6198=CARTESIAN_POINT('',(12.9357864376,-32.5,20.)) ;
#6199=CARTESIAN_POINT('',(1.7763568394E-14,-32.5,20.)) ;
#6200=CARTESIAN_POINT('',(13.2186291507794,-32.3828427117976,20.0000000000016)) ;
#6201=CARTESIAN_POINT('Origin',(12.9357864376,-32.1,20.)) ;
#6202=CARTESIAN_POINT('',(26.7328427125,-18.8686291501,20.)) ;
#6203=CARTESIAN_POINT('',(19.9757359313,-25.6257359313,20.)) ;
#6204=CARTESIAN_POINT('',(27.8642135616524,-18.4,20.)) ;
#6205=CARTESIAN_POINT('Origin',(27.8642135624,-20.,20.)) ;
#6206=CARTESIAN_POINT('',(41.82,-18.4,20.)) ;
#6207=CARTESIAN_POINT('',(34.8421067812,-18.4,20.)) ;
#6208=CARTESIAN_POINT('',(41.85,-18.3699999993067,20.)) ;
#6209=CARTESIAN_POINT('Origin',(41.82,-18.37,20.)) ;
#6210=CARTESIAN_POINT('',(41.85,-10.085,20.)) ;
#6211=CARTESIAN_POINT('Origin',(-41.82,-18.37,19.0299999999991)) ;
#6212=CARTESIAN_POINT('',(-42.45,-18.37,19.4)) ;
#6213=CARTESIAN_POINT('',(-42.15,-18.37,19.7)) ;
#6214=CARTESIAN_POINT('',(-41.82,-19.,19.4)) ;
#6215=CARTESIAN_POINT('Origin',(-41.82,-18.37,19.4)) ;
#6216=CARTESIAN_POINT('',(-41.82,-18.7,19.7)) ;
#6217=CARTESIAN_POINT('Origin',(59.43,-19.,19.4)) ;
#6218=CARTESIAN_POINT('',(-27.8642135624,-19.,19.4)) ;
#6219=CARTESIAN_POINT('',(0.,-19.,19.4)) ;
#6220=CARTESIAN_POINT('',(-27.8642135624,-18.7,19.7)) ;
#6221=CARTESIAN_POINT('Origin',(-27.8642135624,-20.,19.4000000000009)) ;
#6222=CARTESIAN_POINT('',(-27.1571067812,-19.2928932188,19.4)) ;
#6223=CARTESIAN_POINT('Origin',(-27.8642135624,-20.,19.4)) ;
#6224=CARTESIAN_POINT('',(-26.9449747468,-19.0807611845,19.7)) ;
#6225=CARTESIAN_POINT('Origin',(-13.6428932188,-32.8071067812,19.4)) ;
#6226=CARTESIAN_POINT('',(-13.6428932188,-32.8071067812,19.4)) ;
#6227=CARTESIAN_POINT('',(-32.0643145751,-14.3856854249,19.4)) ;
#6228=CARTESIAN_POINT('',(-13.4307611845,-32.5949747468,19.7)) ;
#6229=CARTESIAN_POINT('Origin',(-12.9357864376,-32.1,19.3999999999991)) ;
#6230=CARTESIAN_POINT('',(-12.9357864376,-33.1,19.4)) ;
#6231=CARTESIAN_POINT('Origin',(-12.9357864376,-32.1,19.4)) ;
#6232=CARTESIAN_POINT('',(-12.9357864376,-32.8,19.7)) ;
#6233=CARTESIAN_POINT('Origin',(59.43,-33.1,19.4)) ;
#6234=CARTESIAN_POINT('',(12.9357864376,-33.1,19.4)) ;
#6235=CARTESIAN_POINT('',(0.,-33.1,19.4)) ;
#6236=CARTESIAN_POINT('',(12.9357864376,-32.8,19.7)) ;
#6237=CARTESIAN_POINT('Origin',(12.9357864376,-32.1,19.3999999999991)) ;
#6238=CARTESIAN_POINT('',(13.6428932188,-32.8071067812,19.4)) ;
#6239=CARTESIAN_POINT('Origin',(12.9357864376,-32.1,19.4)) ;
#6240=CARTESIAN_POINT('',(13.4307611845,-32.5949747468,19.7)) ;
#6241=CARTESIAN_POINT('Origin',(6.66573593129,-39.7842640687,19.4)) ;
#6242=CARTESIAN_POINT('',(27.1571067812,-19.2928932188,19.4)) ;
#6243=CARTESIAN_POINT('',(28.5757359313,-17.8742640687,19.4)) ;
#6244=CARTESIAN_POINT('',(26.9449747468,-19.0807611845,19.7)) ;
#6245=CARTESIAN_POINT('Origin',(27.8642135624,-20.,19.4000000000009)) ;
#6246=CARTESIAN_POINT('',(27.8642135624,-19.,19.4)) ;
#6247=CARTESIAN_POINT('Origin',(27.8642135624,-20.,19.4)) ;
#6248=CARTESIAN_POINT('',(27.8642135624,-18.7,19.7)) ;
#6249=CARTESIAN_POINT('Origin',(59.43,-19.,19.4)) ;
#6250=CARTESIAN_POINT('',(41.82,-19.,19.4)) ;
#6251=CARTESIAN_POINT('',(43.6471067812,-19.,19.4)) ;
#6252=CARTESIAN_POINT('',(41.82,-18.7,19.7)) ;
#6253=CARTESIAN_POINT('Origin',(41.82,-18.37,19.0299999999991)) ;
#6254=CARTESIAN_POINT('',(42.45,-18.37,19.4)) ;
#6255=CARTESIAN_POINT('Origin',(41.82,-18.37,19.4)) ;
#6256=CARTESIAN_POINT('',(42.15,-18.37,19.7)) ;
#6257=CARTESIAN_POINT('Origin',(42.45,-39.36,19.4)) ;
#6258=CARTESIAN_POINT('',(42.45,-1.8,19.4)) ;
#6259=CARTESIAN_POINT('',(42.45,-17.45,19.4)) ;
#6260=CARTESIAN_POINT('',(42.15,-1.8,19.7)) ;
#6261=CARTESIAN_POINT('Origin',(-42.45,-39.36,19.4)) ;
#6262=CARTESIAN_POINT('',(-42.45,-1.8,19.4)) ;
#6263=CARTESIAN_POINT('',(-42.15,-1.8,19.7)) ;
#6264=CARTESIAN_POINT('',(-42.45,-17.45,19.4)) ;
#6265=CARTESIAN_POINT('Origin',(0.,0.,-20.)) ;
#6266=CARTESIAN_POINT('',(41.85,-18.3699989753,-20.)) ;
#6267=CARTESIAN_POINT('',(41.85,-1.8,-20.)) ;
#6268=CARTESIAN_POINT('',(41.85,-10.085,-20.)) ;
#6269=CARTESIAN_POINT('',(41.82,-18.4,-20.)) ;
#6270=CARTESIAN_POINT('Origin',(41.82,-18.37,-20.)) ;
#6271=CARTESIAN_POINT('',(27.8642134654,-18.4,-20.)) ;
#6272=CARTESIAN_POINT('',(34.8421067812,-18.4,-20.)) ;
#6273=CARTESIAN_POINT('',(26.7328427125,-18.8686291501,-20.)) ;
#6274=CARTESIAN_POINT('Origin',(27.8642135624,-20.,-20.)) ;
#6275=CARTESIAN_POINT('',(13.2186291611,-32.3828427015,-20.)) ;
#6276=CARTESIAN_POINT('',(19.9757359313,-25.6257359313,-20.)) ;
#6277=CARTESIAN_POINT('',(12.9357864376,-32.5,-20.)) ;
#6278=CARTESIAN_POINT('Origin',(12.9357864376,-32.1,-20.)) ;
#6279=CARTESIAN_POINT('',(-12.9357864376,-32.5,-20.)) ;
#6280=CARTESIAN_POINT('',(2.6645352591E-14,-32.5,-20.)) ;
#6281=CARTESIAN_POINT('',(-13.2186291495519,-32.382842713025,-20.0000000000016)) ;
#6282=CARTESIAN_POINT('Origin',(-12.9357864376,-32.1,-20.)) ;
#6283=CARTESIAN_POINT('',(-26.7328427125,-18.8686291501,-20.)) ;
#6284=CARTESIAN_POINT('',(-19.9757359313,-25.6257359313,-20.)) ;
#6285=CARTESIAN_POINT('',(-27.8642135633724,-18.4,-20.)) ;
#6286=CARTESIAN_POINT('Origin',(-27.8642135624,-20.,-20.)) ;
#6287=CARTESIAN_POINT('',(-41.82,-18.4,-20.)) ;
#6288=CARTESIAN_POINT('',(-34.8421067812,-18.4,-20.)) ;
#6289=CARTESIAN_POINT('',(-41.85,-18.3699991048,-20.)) ;
#6290=CARTESIAN_POINT('Origin',(-41.82,-18.37,-20.)) ;
#6291=CARTESIAN_POINT('',(-41.85,-1.8,-20.)) ;
#6292=CARTESIAN_POINT('',(-41.85,-10.085,-20.)) ;
#6293=CARTESIAN_POINT('',(-35.1465505484,-1.8,-20.)) ;
#6294=CARTESIAN_POINT('',(35.1465505484,-1.8,-20.)) ;
#6295=CARTESIAN_POINT('Origin',(27.8642135624,-20.,0.)) ;
#6296=CARTESIAN_POINT('',(27.1571067812,-19.2928932188,-19.4)) ;
#6297=CARTESIAN_POINT('',(27.8642135323302,-19.,-19.4)) ;
#6298=CARTESIAN_POINT('Origin',(27.8642135624,-20.,-19.4)) ;
#6299=CARTESIAN_POINT('',(27.8642135624,-19.,0.)) ;
#6300=CARTESIAN_POINT('',(27.1571067812,-19.2928932188,0.)) ;
#6301=CARTESIAN_POINT('Origin',(-12.9357864376,-32.1,0.)) ;
#6302=CARTESIAN_POINT('',(-12.9357864376,-33.1,-19.4)) ;
#6303=CARTESIAN_POINT('',(-12.9357864376,-33.1,0.)) ;
#6304=CARTESIAN_POINT('',(-13.6428932188,-32.8071067812,-19.4)) ;
#6305=CARTESIAN_POINT('',(-13.6428932188,-32.8071067812,0.)) ;
#6306=CARTESIAN_POINT('Origin',(-12.9357864376,-32.1,-19.4)) ;
#6307=CARTESIAN_POINT('Origin',(-27.45,-19.,0.)) ;
#6308=CARTESIAN_POINT('',(-27.1571067812,-19.2928932188,-19.4)) ;
#6309=CARTESIAN_POINT('',(-27.1571067812,-19.2928932188,0.)) ;
#6310=CARTESIAN_POINT('',(-20.4,-26.05,-19.4)) ;
#6311=CARTESIAN_POINT('Origin',(27.45,-19.,0.)) ;
#6312=CARTESIAN_POINT('',(13.6428932324447,-32.8071067675488,-19.4000000000025)) ;
#6313=CARTESIAN_POINT('',(20.4,-26.05,-19.4)) ;
#6314=CARTESIAN_POINT('',(13.6428932188,-32.8071067812,0.)) ;
#6315=CARTESIAN_POINT('Origin',(12.9357864376,-32.1,0.)) ;
#6316=CARTESIAN_POINT('',(12.9357864376,-33.1,-19.4)) ;
#6317=CARTESIAN_POINT('',(12.9357864376,-33.1,0.)) ;
#6318=CARTESIAN_POINT('Origin',(12.9357864376,-32.1,-19.4)) ;
#6319=CARTESIAN_POINT('Origin',(-13.35,-33.1,0.)) ;
#6320=CARTESIAN_POINT('',(1.06581410364E-14,-33.1,-19.4)) ;
#6321=CARTESIAN_POINT('Origin',(-27.8642135624,-20.,0.)) ;
#6322=CARTESIAN_POINT('',(-27.8642135624,-19.,-19.4)) ;
#6323=CARTESIAN_POINT('Origin',(-27.8642135624,-20.,-19.4)) ;
#6324=CARTESIAN_POINT('',(-27.8642135624,-19.,0.)) ;
#6325=CARTESIAN_POINT('Origin',(-27.4410276775,-1.8,0.)) ;
#6326=CARTESIAN_POINT('',(42.45,-1.8,-19.4)) ;
#6327=CARTESIAN_POINT('',(42.45,-1.8,0.)) ;
#6328=CARTESIAN_POINT('',(42.15,-1.8,-19.7)) ;
#6329=CARTESIAN_POINT('',(32.1478566738563,-1.8,11.5581330004637)) ;
#6330=CARTESIAN_POINT('Origin',(35.,-1.8,10.)) ;
#6331=CARTESIAN_POINT('',(32.1478566738563,-1.8,-8.44186699953634)) ;
#6332=CARTESIAN_POINT('Origin',(35.,-1.8,-10.)) ;
#6333=CARTESIAN_POINT('Origin',(-27.4410276775,-1.8,0.)) ;
#6334=CARTESIAN_POINT('',(-42.45,-1.8,-19.4)) ;
#6335=CARTESIAN_POINT('',(-42.45,-1.8,0.)) ;
#6336=CARTESIAN_POINT('',(-42.15,-1.8,-19.7)) ;
#6337=CARTESIAN_POINT('',(-37.8521433261437,-1.8,-8.44186699953634)) ;
#6338=CARTESIAN_POINT('Origin',(-35.,-1.8,-10.)) ;
#6339=CARTESIAN_POINT('',(-37.8521433261437,-1.8,11.5581330004637)) ;
#6340=CARTESIAN_POINT('Origin',(-35.,-1.8,10.)) ;
#6341=CARTESIAN_POINT('Origin',(42.45,-1.8,0.)) ;
#6342=CARTESIAN_POINT('',(42.449999999864,-18.3699892404226,-19.4000000000257)) ;
#6343=CARTESIAN_POINT('',(42.45,-10.085,-19.4)) ;
#6344=CARTESIAN_POINT('',(42.45,-18.37,0.)) ;
#6345=CARTESIAN_POINT('Origin',(41.82,-18.37,0.)) ;
#6346=CARTESIAN_POINT('',(41.82,-19.,-19.4)) ;
#6347=CARTESIAN_POINT('',(41.82,-19.,0.)) ;
#6348=CARTESIAN_POINT('Origin',(41.82,-18.37,-19.4)) ;
#6349=CARTESIAN_POINT('Origin',(-42.45,-1.8,0.)) ;
#6350=CARTESIAN_POINT('',(-42.4499999999024,-18.3699906000849,-19.4000000000289)) ;
#6351=CARTESIAN_POINT('',(-42.45,-18.37,0.)) ;
#6352=CARTESIAN_POINT('',(-42.45,-10.085,-19.4)) ;
#6353=CARTESIAN_POINT('Origin',(-41.82,-18.37,0.)) ;
#6354=CARTESIAN_POINT('',(-41.82,-19.,-19.4)) ;
#6355=CARTESIAN_POINT('',(-41.82,-19.,0.)) ;
#6356=CARTESIAN_POINT('Origin',(-41.82,-18.37,-19.4)) ;
#6357=CARTESIAN_POINT('Origin',(-41.82,-18.37,-19.0299999999991)) ;
#6358=CARTESIAN_POINT('',(-42.1499999999,-18.3699901523,-19.7)) ;
#6359=CARTESIAN_POINT('',(-41.82,-18.7,-19.7)) ;
#6360=CARTESIAN_POINT('Origin',(59.43,-19.,-19.4)) ;
#6361=CARTESIAN_POINT('',(-27.8642135624,-18.7,-19.7)) ;
#6362=CARTESIAN_POINT('',(7.1054273576E-15,-19.,-19.4)) ;
#6363=CARTESIAN_POINT('Origin',(-27.8642135624,-20.,-19.4000000000009)) ;
#6364=CARTESIAN_POINT('',(-26.9449747468,-19.0807611845,-19.7)) ;
#6365=CARTESIAN_POINT('Origin',(-6.66573593129,-39.7842640687,-19.4)) ;
#6366=CARTESIAN_POINT('',(-13.4307611845,-32.5949747468,-19.7)) ;
#6367=CARTESIAN_POINT('Origin',(-12.9357864376,-32.1,-19.3999999999991)) ;
#6368=CARTESIAN_POINT('',(-12.9357864376,-32.8,-19.7)) ;
#6369=CARTESIAN_POINT('Origin',(59.43,-33.1,-19.4)) ;
#6370=CARTESIAN_POINT('',(12.9357864376,-32.8,-19.7)) ;
#6371=CARTESIAN_POINT('Origin',(12.9357864376,-32.1,-19.3999999999991)) ;
#6372=CARTESIAN_POINT('',(13.4307612037,-32.5949747276,-19.7)) ;
#6373=CARTESIAN_POINT('Origin',(6.66573593129,-39.7842640687,-19.4)) ;
#6374=CARTESIAN_POINT('',(26.9449747468,-19.0807611845,-19.7)) ;
#6375=CARTESIAN_POINT('Origin',(27.8642135624,-20.,-19.4000000000009)) ;
#6376=CARTESIAN_POINT('',(27.8642134836,-18.7,-19.7)) ;
#6377=CARTESIAN_POINT('Origin',(59.43,-19.,-19.4)) ;
#6378=CARTESIAN_POINT('',(41.82,-18.7,-19.7)) ;
#6379=CARTESIAN_POINT('',(43.6471067812,-19.,-19.4)) ;
#6380=CARTESIAN_POINT('Origin',(41.82,-18.37,-19.0299999999991)) ;
#6381=CARTESIAN_POINT('',(42.1499999998,-18.3699887279,-19.7)) ;
#6382=CARTESIAN_POINT('Origin',(42.45,-39.36,-19.4)) ;
#6383=CARTESIAN_POINT('Origin',(-42.45,-39.36,-19.4)) ;
#6384=CARTESIAN_POINT('Origin',(-35.,-18.9,10.)) ;
#6385=CARTESIAN_POINT('',(-32.3636514836019,-18.4999999999988,8.09942995391034)) ;
#6386=CARTESIAN_POINT('',(-37.8521433261437,-18.5,11.5581330004637)) ;
#6387=CARTESIAN_POINT('Origin',(-35.,-18.5,10.)) ;
#6388=CARTESIAN_POINT('',(-37.8521433261437,-18.9,11.5581330004637)) ;
#6389=CARTESIAN_POINT('Origin',(-35.,-18.5,10.)) ;
#6390=CARTESIAN_POINT('Origin',(-35.,-16.2499999999989,10.0000000000003)) ;
#6391=CARTESIAN_POINT('',(-31.9580594041556,-18.9999999999991,7.80703456220392)) ;
#6392=CARTESIAN_POINT('',(-34.1888158411087,-16.2499999999991,9.4152092165881)) ;
#6393=CARTESIAN_POINT('Origin',(-35.,-19.,10.)) ;
#6394=CARTESIAN_POINT('Origin',(-35.,-18.9,-10.)) ;
#6395=CARTESIAN_POINT('',(-32.363651483595,-18.4999999999987,-11.9005700460802)) ;
#6396=CARTESIAN_POINT('',(-37.8521433261437,-18.5,-8.44186699953634)) ;
#6397=CARTESIAN_POINT('Origin',(-35.,-18.5,-10.)) ;
#6398=CARTESIAN_POINT('',(-37.8521433261437,-18.9,-8.44186699953634)) ;
#6399=CARTESIAN_POINT('Origin',(-35.,-18.5,-10.)) ;
#6400=CARTESIAN_POINT('Origin',(-42.45,-19.,0.)) ;
#6401=CARTESIAN_POINT('',(-31.958059404148,-18.9999999999985,-12.1929654377848)) ;
#6402=CARTESIAN_POINT('Origin',(-35.,-19.,-10.)) ;
#6403=CARTESIAN_POINT('Origin',(-35.,-16.2499999999989,-9.99999999999968)) ;
#6404=CARTESIAN_POINT('',(-34.1888158411066,-16.2499999999991,-10.584790783409)) ;
#6405=CARTESIAN_POINT('Origin',(35.,-18.9,-10.)) ;
#6406=CARTESIAN_POINT('',(37.6363485163993,-18.4999999999987,-11.9005700460881)) ;
#6407=CARTESIAN_POINT('',(32.1478566738563,-18.5,-8.44186699953634)) ;
#6408=CARTESIAN_POINT('Origin',(35.,-18.5,-10.)) ;
#6409=CARTESIAN_POINT('',(32.1478566738563,-18.9,-8.44186699953634)) ;
#6410=CARTESIAN_POINT('Origin',(35.,-18.5,-10.)) ;
#6411=CARTESIAN_POINT('Origin',(35.,-16.2499999999989,-9.99999999999968)) ;
#6412=CARTESIAN_POINT('',(38.0419405958458,-18.9999999999991,-12.1929654377943)) ;
#6413=CARTESIAN_POINT('',(35.8111841588916,-16.2499999999991,-10.5847907834114)) ;
#6414=CARTESIAN_POINT('Origin',(35.,-19.,-10.)) ;
#6415=CARTESIAN_POINT('Origin',(35.,-18.9,10.)) ;
#6416=CARTESIAN_POINT('',(37.6363485163777,-18.4999999999987,8.09942995388186)) ;
#6417=CARTESIAN_POINT('',(32.1478566738563,-18.5,11.5581330004637)) ;
#6418=CARTESIAN_POINT('Origin',(35.,-18.5,10.)) ;
#6419=CARTESIAN_POINT('',(32.1478566738563,-18.9,11.5581330004637)) ;
#6420=CARTESIAN_POINT('Origin',(35.,-18.5,10.)) ;
#6421=CARTESIAN_POINT('Origin',(-42.45,-19.,0.)) ;
#6422=CARTESIAN_POINT('',(38.0419405958204,-18.9999999999985,7.80703456217137)) ;
#6423=CARTESIAN_POINT('Origin',(35.,-19.,10.)) ;
#6424=CARTESIAN_POINT('Origin',(35.,-16.2499999999989,10.0000000000003)) ;
#6425=CARTESIAN_POINT('',(35.811184158885,-16.2499999999991,9.41520921657933)) ;
#6758=UNCERTAINTY_MEASURE_WITH_UNIT(LENGTH_MEASURE(0.01),#6780,
'DISTANCE_ACCURACY_VALUE',
'Maximum model space distance between geometric entities at asserted c
onnectivities') ;
#6767=UNCERTAINTY_MEASURE_WITH_UNIT(LENGTH_MEASURE(0.01),#6780,
'DISTANCE_ACCURACY_VALUE',
'Maximum model space distance between geometric entities at asserted c
onnectivities') ;
#6770=(
GEOMETRIC_REPRESENTATION_CONTEXT(3)
GLOBAL_UNCERTAINTY_ASSIGNED_CONTEXT((#6758))
GLOBAL_UNIT_ASSIGNED_CONTEXT((#6780,#6782,#6783))
REPRESENTATION_CONTEXT('','3D')
) ;
#6779=(
GEOMETRIC_REPRESENTATION_CONTEXT(3)
GLOBAL_UNCERTAINTY_ASSIGNED_CONTEXT((#6767))
GLOBAL_UNIT_ASSIGNED_CONTEXT((#6780,#6782,#6783))
REPRESENTATION_CONTEXT('','3D')
) ;
#6780=(
LENGTH_UNIT()
NAMED_UNIT(*)
SI_UNIT(.MILLI.,.METRE.)
) ;
#6782=(
NAMED_UNIT(*)
PLANE_ANGLE_UNIT()
SI_UNIT($,.RADIAN.)
) ;
#6783=(
NAMED_UNIT(*)
SI_UNIT($,.STERADIAN.)
SOLID_ANGLE_UNIT()
) ;
#6786=SHAPE_DEFINITION_REPRESENTATION(#6797,#6818) ;
#6797=PRODUCT_DEFINITION_SHAPE('',$,#6830) ;
#6818=SHAPE_REPRESENTATION('',(#4192),#6770) ;
#6827=PRODUCT_DEFINITION_CONTEXT('part definition',#6862,'design') ;
#6830=PRODUCT_DEFINITION('Clamp_Body_Lower','Clamp_Body_Lower',#6841,#6827) ;
#6841=PRODUCT_DEFINITION_FORMATION('',$,#6866) ;
#6862=APPLICATION_CONTEXT(
'Core Data for Automotive Mechanical Design Process') ;
#6863=PRODUCT_CONTEXT('part definition',#6862,'mechanical') ;
#6866=PRODUCT('Clamp_Body_Lower','Clamp_Body_Lower',$,(#6863)) ;
#6876=PRESENTATION_STYLE_ASSIGNMENT((#6879)) ;
#6879=SURFACE_STYLE_USAGE(.BOTH.,#6882) ;
#6882=SURFACE_SIDE_STYLE('',(#6885)) ;
#6885=SURFACE_STYLE_FILL_AREA(#6888) ;
#6888=FILL_AREA_STYLE('Opaque(245,245,246)',(#6891)) ;
#6891=FILL_AREA_STYLE_COLOUR('Opaque(245,245,246)',#6894) ;
#6894=COLOUR_RGB('Opaque(245,245,246)', 0.09019608, 0.27058824, 0.51372549) ;
ENDSEC;
END-ISO-10303-21;
